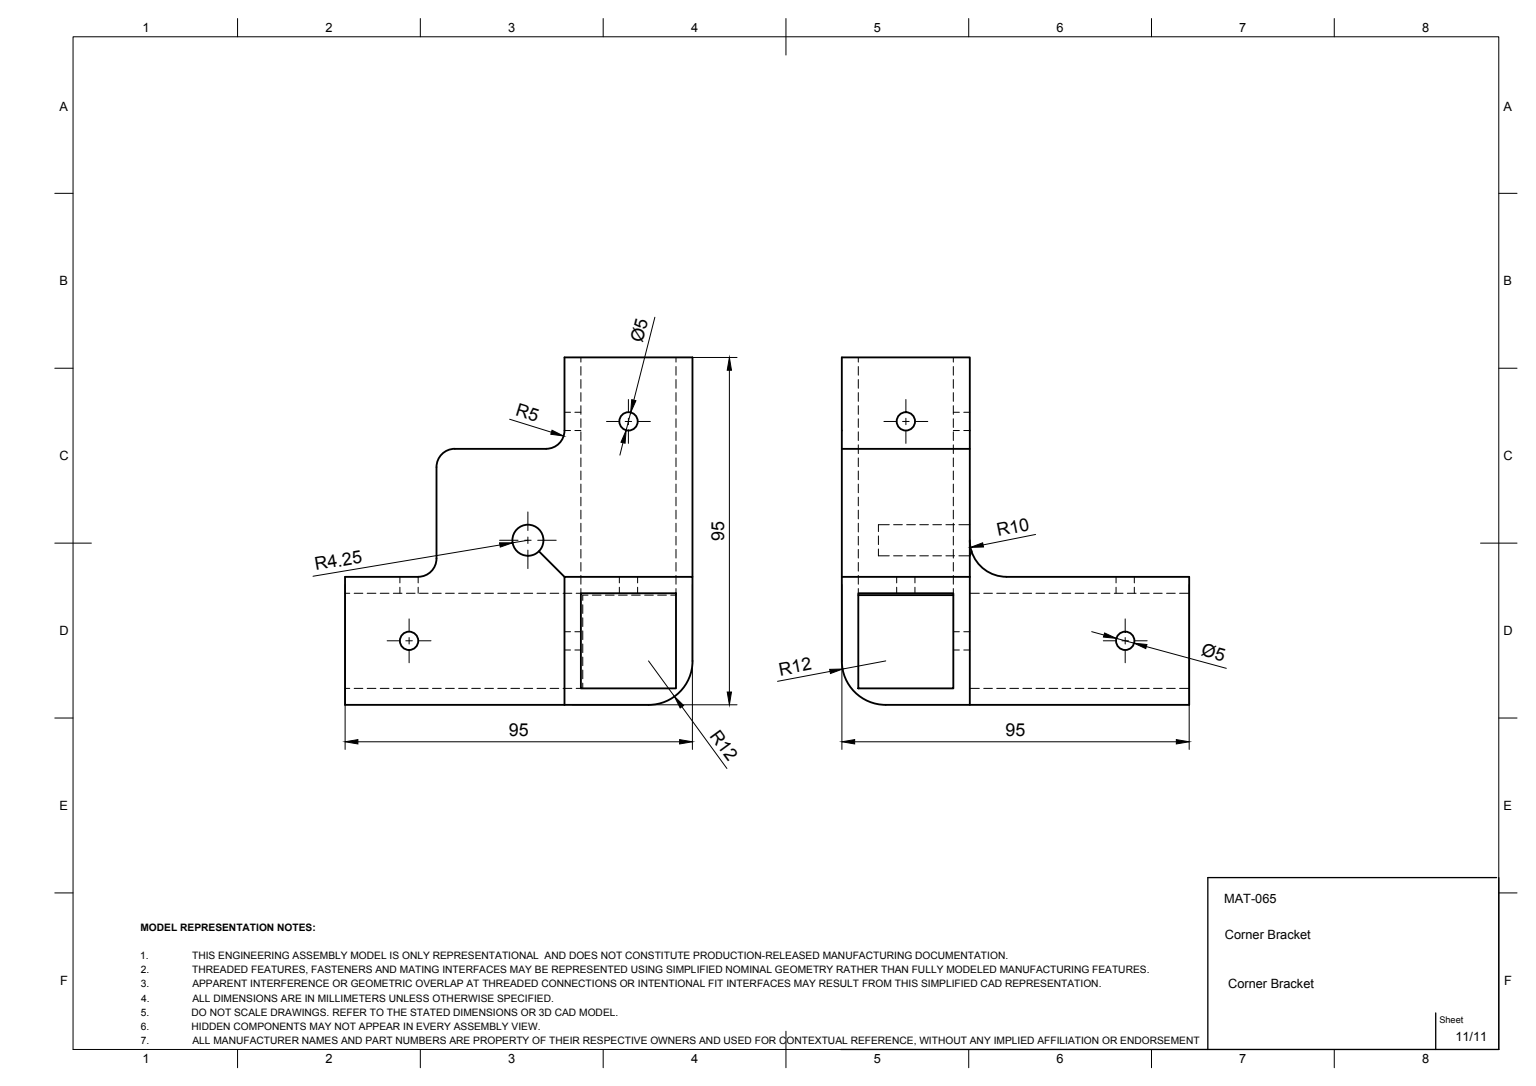
ISO-10303-21;
HEADER;
/* Generated by software containing ST-Developer
 * from STEP Tools, Inc. (www.steptools.com) 
 */

FILE_DESCRIPTION(
/* description */ (
'CAx-IF Rec.Pracs.---Representation and Presentation of Product Manufa
cturing Information (PMI)---4.0---2014-10-13'),
/* implementation_level */ '2;1');

FILE_NAME(
/* name */ 'Corner Bracket.step',
/* time_stamp */ '2026-11-15T23:28:27-08:00',
/* author */ (''),
/* organization */ (''),
/* preprocessor_version */ 'ST-DEVELOPER v20.2',
/* originating_system */ 'Autodesk Translation Framework v15.17.0.0',
/* authorisation */ '');

FILE_SCHEMA (('AUTOMOTIVE_DESIGN { 1 0 10303 214 3 1 1 }'));
ENDSEC;

DATA;
#10=MECHANICAL_DESIGN_GEOMETRIC_PRESENTATION_REPRESENTATION('',(#195),#7756);
#163=SPHERICAL_SURFACE('',#4954,0.012);
#165=ELLIPSE('',#4934,0.0141421356237309,0.01);
#167=B_SPLINE_CURVE_WITH_KNOTS('',3,(#7200,#7201,#7202,#7203,#7204,#7205),
 .UNSPECIFIED.,.F.,.F.,(4,2,4),(-0.973960746358264,-0.811705326326323,-0.649449906294381),
 .UNSPECIFIED.);
#168=B_SPLINE_CURVE_WITH_KNOTS('',3,(#7231,#7232,#7233,#7234,#7235,#7236),
 .UNSPECIFIED.,.F.,.F.,(4,2,4),(0.649449906294381,0.811705326326323,0.973960746358265),
 .UNSPECIFIED.);
#177=SHAPE_REPRESENTATION_RELATIONSHIP('SRR','None',#7825,#186);
#186=ADVANCED_BREP_SHAPE_REPRESENTATION('',(#204),#7753);
#195=STYLED_ITEM('',(#7873),#204);
#204=MANIFOLD_SOLID_BREP('Body1',#4632);
#224=CYLINDRICAL_SURFACE('',#4933,0.01);
#225=CYLINDRICAL_SURFACE('',#4935,0.012);
#226=CYLINDRICAL_SURFACE('',#4937,0.0025);
#227=CYLINDRICAL_SURFACE('',#4938,0.0025);
#228=CYLINDRICAL_SURFACE('',#4939,0.0025);
#229=CYLINDRICAL_SURFACE('',#4940,0.0025);
#230=CYLINDRICAL_SURFACE('',#4941,0.0025);
#231=CYLINDRICAL_SURFACE('',#4942,0.0025);
#232=CYLINDRICAL_SURFACE('',#4945,0.00425);
#233=CYLINDRICAL_SURFACE('',#4948,0.01);
#234=CYLINDRICAL_SURFACE('',#4949,0.005);
#235=CYLINDRICAL_SURFACE('',#4950,0.005);
#236=CYLINDRICAL_SURFACE('',#4951,0.005);
#237=CYLINDRICAL_SURFACE('',#4952,0.012);
#238=CYLINDRICAL_SURFACE('',#4956,0.012);
#298=CIRCLE('',#4884,0.0025);
#299=CIRCLE('',#4885,0.0025);
#300=CIRCLE('',#4887,0.0025);
#301=CIRCLE('',#4888,0.0025);
#302=CIRCLE('',#4890,0.012);
#303=CIRCLE('',#4892,0.012);
#304=CIRCLE('',#4895,0.012);
#305=CIRCLE('',#4897,0.01);
#306=CIRCLE('',#4899,0.01);
#307=CIRCLE('',#4901,0.005);
#308=CIRCLE('',#4902,0.005);
#309=CIRCLE('',#4903,0.00425);
#310=CIRCLE('',#4904,0.005);
#311=CIRCLE('',#4905,0.0025);
#312=CIRCLE('',#4906,0.0025);
#313=CIRCLE('',#4908,0.005);
#314=CIRCLE('',#4909,0.005);
#315=CIRCLE('',#4910,0.005);
#316=CIRCLE('',#4912,0.0025);
#317=CIRCLE('',#4914,0.0025);
#318=CIRCLE('',#4916,0.0025);
#319=CIRCLE('',#4917,0.0025);
#320=CIRCLE('',#4921,0.0025);
#321=CIRCLE('',#4923,0.0025);
#322=CIRCLE('',#4927,0.0025);
#323=CIRCLE('',#4931,0.0025);
#324=CIRCLE('',#4936,0.012);
#325=CIRCLE('',#4946,0.00425);
#326=CIRCLE('',#4953,0.012);
#327=CIRCLE('',#4955,0.012);
#407=FACE_BOUND('',#823,.T.);
#408=FACE_BOUND('',#825,.T.);
#409=FACE_BOUND('',#828,.T.);
#410=FACE_BOUND('',#832,.T.);
#411=FACE_BOUND('',#833,.T.);
#412=FACE_BOUND('',#836,.T.);
#413=FACE_BOUND('',#838,.T.);
#414=FACE_BOUND('',#840,.T.);
#415=FACE_BOUND('',#841,.T.);
#416=FACE_BOUND('',#845,.T.);
#417=FACE_BOUND('',#847,.T.);
#418=FACE_BOUND('',#851,.T.);
#419=FACE_BOUND('',#855,.T.);
#558=FACE_OUTER_BOUND('',#820,.T.);
#559=FACE_OUTER_BOUND('',#821,.T.);
#560=FACE_OUTER_BOUND('',#822,.T.);
#561=FACE_OUTER_BOUND('',#824,.T.);
#562=FACE_OUTER_BOUND('',#826,.T.);
#563=FACE_OUTER_BOUND('',#827,.T.);
#564=FACE_OUTER_BOUND('',#829,.T.);
#565=FACE_OUTER_BOUND('',#830,.T.);
#566=FACE_OUTER_BOUND('',#831,.T.);
#567=FACE_OUTER_BOUND('',#834,.T.);
#568=FACE_OUTER_BOUND('',#835,.T.);
#569=FACE_OUTER_BOUND('',#837,.T.);
#570=FACE_OUTER_BOUND('',#839,.T.);
#571=FACE_OUTER_BOUND('',#842,.T.);
#572=FACE_OUTER_BOUND('',#843,.T.);
#573=FACE_OUTER_BOUND('',#844,.T.);
#574=FACE_OUTER_BOUND('',#846,.T.);
#575=FACE_OUTER_BOUND('',#848,.T.);
#576=FACE_OUTER_BOUND('',#849,.T.);
#577=FACE_OUTER_BOUND('',#850,.T.);
#578=FACE_OUTER_BOUND('',#852,.T.);
#579=FACE_OUTER_BOUND('',#853,.T.);
#580=FACE_OUTER_BOUND('',#854,.T.);
#581=FACE_OUTER_BOUND('',#856,.T.);
#582=FACE_OUTER_BOUND('',#857,.T.);
#583=FACE_OUTER_BOUND('',#858,.T.);
#584=FACE_OUTER_BOUND('',#859,.T.);
#585=FACE_OUTER_BOUND('',#860,.T.);
#586=FACE_OUTER_BOUND('',#861,.T.);
#587=FACE_OUTER_BOUND('',#862,.T.);
#588=FACE_OUTER_BOUND('',#863,.T.);
#589=FACE_OUTER_BOUND('',#864,.T.);
#590=FACE_OUTER_BOUND('',#865,.T.);
#591=FACE_OUTER_BOUND('',#866,.T.);
#592=FACE_OUTER_BOUND('',#867,.T.);
#593=FACE_OUTER_BOUND('',#868,.T.);
#594=FACE_OUTER_BOUND('',#869,.T.);
#595=FACE_OUTER_BOUND('',#870,.T.);
#596=FACE_OUTER_BOUND('',#871,.T.);
#597=FACE_OUTER_BOUND('',#872,.T.);
#598=FACE_OUTER_BOUND('',#873,.T.);
#599=FACE_OUTER_BOUND('',#874,.T.);
#600=FACE_OUTER_BOUND('',#875,.T.);
#820=EDGE_LOOP('',(#3551,#3552,#3553,#3554,#3555,#3556,#3557));
#821=EDGE_LOOP('',(#3558,#3559,#3560,#3561,#3562,#3563,#3564));
#822=EDGE_LOOP('',(#3565,#3566,#3567,#3568,#3569));
#823=EDGE_LOOP('',(#3570,#3571,#3572,#3573));
#824=EDGE_LOOP('',(#3574,#3575,#3576,#3577,#3578));
#825=EDGE_LOOP('',(#3579,#3580,#3581,#3582));
#826=EDGE_LOOP('',(#3583,#3584,#3585,#3586));
#827=EDGE_LOOP('',(#3587,#3588,#3589,#3590,#3591));
#828=EDGE_LOOP('',(#3592,#3593,#3594,#3595));
#829=EDGE_LOOP('',(#3596,#3597,#3598,#3599,#3600,#3601,#3602));
#830=EDGE_LOOP('',(#3603,#3604,#3605,#3606,#3607,#3608,#3609));
#831=EDGE_LOOP('',(#3610,#3611,#3612,#3613,#3614,#3615,#3616,#3617,#3618,
#3619,#3620,#3621,#3622,#3623));
#832=EDGE_LOOP('',(#3624));
#833=EDGE_LOOP('',(#3625));
#834=EDGE_LOOP('',(#3626,#3627,#3628,#3629,#3630,#3631,#3632,#3633,#3634,
#3635,#3636));
#835=EDGE_LOOP('',(#3637,#3638,#3639,#3640));
#836=EDGE_LOOP('',(#3641));
#837=EDGE_LOOP('',(#3642,#3643,#3644,#3645));
#838=EDGE_LOOP('',(#3646));
#839=EDGE_LOOP('',(#3647,#3648,#3649,#3650,#3651,#3652,#3653,#3654));
#840=EDGE_LOOP('',(#3655));
#841=EDGE_LOOP('',(#3656));
#842=EDGE_LOOP('',(#3657,#3658,#3659,#3660));
#843=EDGE_LOOP('',(#3661,#3662,#3663,#3664,#3665,#3666,#3667,#3668));
#844=EDGE_LOOP('',(#3669,#3670,#3671,#3672));
#845=EDGE_LOOP('',(#3673));
#846=EDGE_LOOP('',(#3674,#3675,#3676,#3677));
#847=EDGE_LOOP('',(#3678));
#848=EDGE_LOOP('',(#3679,#3680,#3681,#3682));
#849=EDGE_LOOP('',(#3683,#3684,#3685,#3686));
#850=EDGE_LOOP('',(#3687,#3688,#3689,#3690));
#851=EDGE_LOOP('',(#3691));
#852=EDGE_LOOP('',(#3692,#3693,#3694,#3695));
#853=EDGE_LOOP('',(#3696,#3697,#3698,#3699));
#854=EDGE_LOOP('',(#3700,#3701,#3702,#3703));
#855=EDGE_LOOP('',(#3704));
#856=EDGE_LOOP('',(#3705,#3706,#3707,#3708));
#857=EDGE_LOOP('',(#3709,#3710,#3711,#3712,#3713));
#858=EDGE_LOOP('',(#3714,#3715,#3716,#3717));
#859=EDGE_LOOP('',(#3718,#3719,#3720,#3721));
#860=EDGE_LOOP('',(#3722,#3723,#3724,#3725));
#861=EDGE_LOOP('',(#3726,#3727,#3728,#3729));
#862=EDGE_LOOP('',(#3730,#3731,#3732,#3733,#3734));
#863=EDGE_LOOP('',(#3735,#3736,#3737,#3738));
#864=EDGE_LOOP('',(#3739,#3740,#3741,#3742,#3743));
#865=EDGE_LOOP('',(#3744,#3745,#3746,#3747));
#866=EDGE_LOOP('',(#3748,#3749,#3750,#3751));
#867=EDGE_LOOP('',(#3752,#3753,#3754,#3755,#3756,#3757));
#868=EDGE_LOOP('',(#3758));
#869=EDGE_LOOP('',(#3759,#3760,#3761,#3762,#3763));
#870=EDGE_LOOP('',(#3764,#3765,#3766,#3767,#3768));
#871=EDGE_LOOP('',(#3769,#3770,#3771,#3772,#3773));
#872=EDGE_LOOP('',(#3774,#3775,#3776,#3777));
#873=EDGE_LOOP('',(#3778,#3779,#3780,#3781));
#874=EDGE_LOOP('',(#3782,#3783,#3784));
#875=EDGE_LOOP('',(#3785,#3786,#3787,#3788));
#1237=LINE('',#7001,#1730);
#1238=LINE('',#7003,#1731);
#1239=LINE('',#7008,#1732);
#1240=LINE('',#7010,#1733);
#1241=LINE('',#7011,#1734);
#1242=LINE('',#7015,#1735);
#1243=LINE('',#7017,#1736);
#1244=LINE('',#7022,#1737);
#1245=LINE('',#7024,#1738);
#1246=LINE('',#7025,#1739);
#1247=LINE('',#7029,#1740);
#1248=LINE('',#7033,#1741);
#1249=LINE('',#7035,#1742);
#1250=LINE('',#7036,#1743);
#1251=LINE('',#7039,#1744);
#1252=LINE('',#7041,#1745);
#1253=LINE('',#7043,#1746);
#1254=LINE('',#7044,#1747);
#1255=LINE('',#7047,#1748);
#1256=LINE('',#7051,#1749);
#1257=LINE('',#7052,#1750);
#1258=LINE('',#7055,#1751);
#1259=LINE('',#7057,#1752);
#1260=LINE('',#7059,#1753);
#1261=LINE('',#7060,#1754);
#1262=LINE('',#7064,#1755);
#1263=LINE('',#7066,#1756);
#1264=LINE('',#7068,#1757);
#1265=LINE('',#7069,#1758);
#1266=LINE('',#7073,#1759);
#1267=LINE('',#7076,#1760);
#1268=LINE('',#7077,#1761);
#1269=LINE('',#7080,#1762);
#1270=LINE('',#7082,#1763);
#1271=LINE('',#7084,#1764);
#1272=LINE('',#7085,#1765);
#1273=LINE('',#7088,#1766);
#1274=LINE('',#7089,#1767);
#1275=LINE('',#7091,#1768);
#1276=LINE('',#7094,#1769);
#1277=LINE('',#7097,#1770);
#1278=LINE('',#7098,#1771);
#1279=LINE('',#7100,#1772);
#1280=LINE('',#7103,#1773);
#1281=LINE('',#7107,#1774);
#1282=LINE('',#7111,#1775);
#1283=LINE('',#7114,#1776);
#1284=LINE('',#7117,#1777);
#1285=LINE('',#7125,#1778);
#1286=LINE('',#7126,#1779);
#1287=LINE('',#7130,#1780);
#1288=LINE('',#7134,#1781);
#1289=LINE('',#7138,#1782);
#1290=LINE('',#7139,#1783);
#1291=LINE('',#7143,#1784);
#1292=LINE('',#7148,#1785);
#1293=LINE('',#7149,#1786);
#1294=LINE('',#7151,#1787);
#1295=LINE('',#7152,#1788);
#1296=LINE('',#7153,#1789);
#1297=LINE('',#7159,#1790);
#1298=LINE('',#7162,#1791);
#1299=LINE('',#7163,#1792);
#1300=LINE('',#7165,#1793);
#1301=LINE('',#7166,#1794);
#1302=LINE('',#7168,#1795);
#1303=LINE('',#7175,#1796);
#1304=LINE('',#7179,#1797);
#1305=LINE('',#7181,#1798);
#1306=LINE('',#7182,#1799);
#1307=LINE('',#7187,#1800);
#1308=LINE('',#7188,#1801);
#1309=LINE('',#7191,#1802);
#1310=LINE('',#7192,#1803);
#1311=LINE('',#7194,#1804);
#1312=LINE('',#7210,#1805);
#1313=LINE('',#7212,#1806);
#1314=LINE('',#7214,#1807);
#1315=LINE('',#7216,#1808);
#1316=LINE('',#7218,#1809);
#1317=LINE('',#7220,#1810);
#1318=LINE('',#7222,#1811);
#1319=LINE('',#7223,#1812);
#1320=LINE('',#7225,#1813);
#1321=LINE('',#7226,#1814);
#1322=LINE('',#7230,#1815);
#1730=VECTOR('',#5675,1.);
#1731=VECTOR('',#5676,1.);
#1732=VECTOR('',#5681,1.);
#1733=VECTOR('',#5682,1.);
#1734=VECTOR('',#5683,1.);
#1735=VECTOR('',#5686,1.);
#1736=VECTOR('',#5687,1.);
#1737=VECTOR('',#5692,1.);
#1738=VECTOR('',#5693,1.);
#1739=VECTOR('',#5694,1.);
#1740=VECTOR('',#5697,1.);
#1741=VECTOR('',#5700,1.);
#1742=VECTOR('',#5701,1.);
#1743=VECTOR('',#5702,1.);
#1744=VECTOR('',#5703,1.);
#1745=VECTOR('',#5704,1.);
#1746=VECTOR('',#5705,1.);
#1747=VECTOR('',#5706,1.);
#1748=VECTOR('',#5709,1.);
#1749=VECTOR('',#5712,1.);
#1750=VECTOR('',#5713,1.);
#1751=VECTOR('',#5714,1.);
#1752=VECTOR('',#5715,1.);
#1753=VECTOR('',#5716,1.);
#1754=VECTOR('',#5717,1.);
#1755=VECTOR('',#5720,1.);
#1756=VECTOR('',#5721,1.);
#1757=VECTOR('',#5722,1.);
#1758=VECTOR('',#5723,1.);
#1759=VECTOR('',#5726,1.);
#1760=VECTOR('',#5729,1.);
#1761=VECTOR('',#5730,1.);
#1762=VECTOR('',#5731,1.);
#1763=VECTOR('',#5732,1.);
#1764=VECTOR('',#5733,1.);
#1765=VECTOR('',#5734,1.);
#1766=VECTOR('',#5737,1.);
#1767=VECTOR('',#5738,1.);
#1768=VECTOR('',#5739,1.);
#1769=VECTOR('',#5742,1.);
#1770=VECTOR('',#5745,1.);
#1771=VECTOR('',#5746,1.);
#1772=VECTOR('',#5747,1.);
#1773=VECTOR('',#5750,1.);
#1774=VECTOR('',#5753,1.);
#1775=VECTOR('',#5756,1.);
#1776=VECTOR('',#5759,1.);
#1777=VECTOR('',#5762,1.);
#1778=VECTOR('',#5771,1.);
#1779=VECTOR('',#5772,1.);
#1780=VECTOR('',#5775,1.);
#1781=VECTOR('',#5778,1.);
#1782=VECTOR('',#5783,1.);
#1783=VECTOR('',#5784,1.);
#1784=VECTOR('',#5789,1.);
#1785=VECTOR('',#5794,1.);
#1786=VECTOR('',#5795,1.);
#1787=VECTOR('',#5796,1.);
#1788=VECTOR('',#5797,1.);
#1789=VECTOR('',#5798,1.);
#1790=VECTOR('',#5805,1.);
#1791=VECTOR('',#5808,1.);
#1792=VECTOR('',#5809,1.);
#1793=VECTOR('',#5810,1.);
#1794=VECTOR('',#5811,1.);
#1795=VECTOR('',#5814,1.);
#1796=VECTOR('',#5823,1.);
#1797=VECTOR('',#5828,1.);
#1798=VECTOR('',#5829,1.);
#1799=VECTOR('',#5830,1.);
#1800=VECTOR('',#5835,1.);
#1801=VECTOR('',#5836,1.);
#1802=VECTOR('',#5839,1.);
#1803=VECTOR('',#5840,1.);
#1804=VECTOR('',#5843,1.);
#1805=VECTOR('',#5858,0.0025);
#1806=VECTOR('',#5861,0.0025);
#1807=VECTOR('',#5864,0.0025);
#1808=VECTOR('',#5867,0.0025);
#1809=VECTOR('',#5870,0.0025);
#1810=VECTOR('',#5873,0.0025);
#1811=VECTOR('',#5876,1.);
#1812=VECTOR('',#5877,1.);
#1813=VECTOR('',#5880,1.);
#1814=VECTOR('',#5881,1.);
#1815=VECTOR('',#5886,0.00425);
#2164=VERTEX_POINT('',#6999);
#2165=VERTEX_POINT('',#7000);
#2166=VERTEX_POINT('',#7002);
#2167=VERTEX_POINT('',#7004);
#2168=VERTEX_POINT('',#7007);
#2169=VERTEX_POINT('',#7009);
#2170=VERTEX_POINT('',#7013);
#2171=VERTEX_POINT('',#7014);
#2172=VERTEX_POINT('',#7016);
#2173=VERTEX_POINT('',#7018);
#2174=VERTEX_POINT('',#7021);
#2175=VERTEX_POINT('',#7023);
#2176=VERTEX_POINT('',#7027);
#2177=VERTEX_POINT('',#7028);
#2178=VERTEX_POINT('',#7030);
#2179=VERTEX_POINT('',#7032);
#2180=VERTEX_POINT('',#7034);
#2181=VERTEX_POINT('',#7037);
#2182=VERTEX_POINT('',#7038);
#2183=VERTEX_POINT('',#7040);
#2184=VERTEX_POINT('',#7042);
#2185=VERTEX_POINT('',#7046);
#2186=VERTEX_POINT('',#7048);
#2187=VERTEX_POINT('',#7050);
#2188=VERTEX_POINT('',#7053);
#2189=VERTEX_POINT('',#7054);
#2190=VERTEX_POINT('',#7056);
#2191=VERTEX_POINT('',#7058);
#2192=VERTEX_POINT('',#7062);
#2193=VERTEX_POINT('',#7063);
#2194=VERTEX_POINT('',#7065);
#2195=VERTEX_POINT('',#7067);
#2196=VERTEX_POINT('',#7071);
#2197=VERTEX_POINT('',#7072);
#2198=VERTEX_POINT('',#7074);
#2199=VERTEX_POINT('',#7078);
#2200=VERTEX_POINT('',#7079);
#2201=VERTEX_POINT('',#7081);
#2202=VERTEX_POINT('',#7083);
#2203=VERTEX_POINT('',#7087);
#2204=VERTEX_POINT('',#7090);
#2205=VERTEX_POINT('',#7092);
#2206=VERTEX_POINT('',#7096);
#2207=VERTEX_POINT('',#7099);
#2208=VERTEX_POINT('',#7101);
#2209=VERTEX_POINT('',#7105);
#2210=VERTEX_POINT('',#7106);
#2211=VERTEX_POINT('',#7108);
#2212=VERTEX_POINT('',#7110);
#2213=VERTEX_POINT('',#7113);
#2214=VERTEX_POINT('',#7115);
#2215=VERTEX_POINT('',#7119);
#2216=VERTEX_POINT('',#7121);
#2217=VERTEX_POINT('',#7124);
#2218=VERTEX_POINT('',#7127);
#2219=VERTEX_POINT('',#7129);
#2220=VERTEX_POINT('',#7131);
#2221=VERTEX_POINT('',#7133);
#2222=VERTEX_POINT('',#7137);
#2223=VERTEX_POINT('',#7140);
#2224=VERTEX_POINT('',#7144);
#2225=VERTEX_POINT('',#7147);
#2226=VERTEX_POINT('',#7150);
#2227=VERTEX_POINT('',#7154);
#2228=VERTEX_POINT('',#7156);
#2229=VERTEX_POINT('',#7161);
#2230=VERTEX_POINT('',#7164);
#2231=VERTEX_POINT('',#7169);
#2232=VERTEX_POINT('',#7172);
#2233=VERTEX_POINT('',#7178);
#2234=VERTEX_POINT('',#7180);
#2235=VERTEX_POINT('',#7183);
#2236=VERTEX_POINT('',#7186);
#2237=VERTEX_POINT('',#7190);
#2238=VERTEX_POINT('',#7195);
#2239=VERTEX_POINT('',#7199);
#2240=VERTEX_POINT('',#7228);
#2659=EDGE_CURVE('',#2164,#2165,#1237,.T.);
#2660=EDGE_CURVE('',#2165,#2166,#1238,.T.);
#2661=EDGE_CURVE('',#2167,#2166,#298,.T.);
#2662=EDGE_CURVE('',#2166,#2167,#299,.T.);
#2663=EDGE_CURVE('',#2166,#2168,#1239,.T.);
#2664=EDGE_CURVE('',#2169,#2168,#1240,.T.);
#2665=EDGE_CURVE('',#2164,#2169,#1241,.T.);
#2666=EDGE_CURVE('',#2170,#2171,#1242,.T.);
#2667=EDGE_CURVE('',#2170,#2172,#1243,.F.);
#2668=EDGE_CURVE('',#2173,#2172,#300,.T.);
#2669=EDGE_CURVE('',#2172,#2173,#301,.T.);
#2670=EDGE_CURVE('',#2172,#2174,#1244,.F.);
#2671=EDGE_CURVE('',#2174,#2175,#1245,.T.);
#2672=EDGE_CURVE('',#2175,#2171,#1246,.T.);
#2673=EDGE_CURVE('',#2176,#2177,#1247,.T.);
#2674=EDGE_CURVE('',#2177,#2178,#302,.T.);
#2675=EDGE_CURVE('',#2178,#2179,#1248,.T.);
#2676=EDGE_CURVE('',#2180,#2179,#1249,.T.);
#2677=EDGE_CURVE('',#2180,#2176,#1250,.T.);
#2678=EDGE_CURVE('',#2181,#2182,#1251,.T.);
#2679=EDGE_CURVE('',#2181,#2183,#1252,.T.);
#2680=EDGE_CURVE('',#2183,#2184,#1253,.T.);
#2681=EDGE_CURVE('',#2182,#2184,#1254,.T.);
#2682=EDGE_CURVE('',#2185,#2169,#1255,.T.);
#2683=EDGE_CURVE('',#2185,#2186,#303,.T.);
#2684=EDGE_CURVE('',#2187,#2186,#1256,.T.);
#2685=EDGE_CURVE('',#2187,#2164,#1257,.T.);
#2686=EDGE_CURVE('',#2188,#2189,#1258,.T.);
#2687=EDGE_CURVE('',#2188,#2190,#1259,.T.);
#2688=EDGE_CURVE('',#2190,#2191,#1260,.T.);
#2689=EDGE_CURVE('',#2189,#2191,#1261,.T.);
#2690=EDGE_CURVE('',#2192,#2193,#1262,.T.);
#2691=EDGE_CURVE('',#2193,#2194,#1263,.T.);
#2692=EDGE_CURVE('',#2195,#2194,#1264,.T.);
#2693=EDGE_CURVE('',#2195,#2192,#1265,.T.);
#2694=EDGE_CURVE('',#2196,#2197,#1266,.T.);
#2695=EDGE_CURVE('',#2197,#2198,#304,.T.);
#2696=EDGE_CURVE('',#2171,#2198,#1267,.T.);
#2697=EDGE_CURVE('',#2175,#2196,#1268,.T.);
#2698=EDGE_CURVE('',#2199,#2200,#1269,.T.);
#2699=EDGE_CURVE('',#2199,#2201,#1270,.T.);
#2700=EDGE_CURVE('',#2201,#2202,#1271,.T.);
#2701=EDGE_CURVE('',#2200,#2202,#1272,.T.);
#2702=EDGE_CURVE('',#2186,#2203,#1273,.T.);
#2703=EDGE_CURVE('',#2203,#2177,#1274,.F.);
#2704=EDGE_CURVE('',#2176,#2204,#1275,.T.);
#2705=EDGE_CURVE('',#2204,#2205,#305,.T.);
#2706=EDGE_CURVE('',#2187,#2205,#1276,.T.);
#2707=EDGE_CURVE('',#2178,#2206,#1277,.T.);
#2708=EDGE_CURVE('',#2206,#2197,#1278,.T.);
#2709=EDGE_CURVE('',#2207,#2196,#1279,.T.);
#2710=EDGE_CURVE('',#2207,#2208,#306,.T.);
#2711=EDGE_CURVE('',#2179,#2208,#1280,.T.);
#2712=EDGE_CURVE('',#2209,#2210,#1281,.T.);
#2713=EDGE_CURVE('',#2209,#2211,#307,.T.);
#2714=EDGE_CURVE('',#2211,#2212,#1282,.T.);
#2715=EDGE_CURVE('',#2212,#2165,#308,.F.);
#2716=EDGE_CURVE('',#2205,#2213,#1283,.F.);
#2717=EDGE_CURVE('',#2214,#2213,#309,.T.);
#2718=EDGE_CURVE('',#2214,#2207,#1284,.T.);
#2719=EDGE_CURVE('',#2174,#2210,#310,.F.);
#2720=EDGE_CURVE('',#2215,#2215,#311,.T.);
#2721=EDGE_CURVE('',#2216,#2216,#312,.T.);
#2722=EDGE_CURVE('',#2198,#2217,#1285,.F.);
#2723=EDGE_CURVE('',#2217,#2185,#1286,.F.);
#2724=EDGE_CURVE('',#2168,#2218,#313,.T.);
#2725=EDGE_CURVE('',#2219,#2218,#1287,.T.);
#2726=EDGE_CURVE('',#2219,#2220,#314,.F.);
#2727=EDGE_CURVE('',#2220,#2221,#1288,.T.);
#2728=EDGE_CURVE('',#2221,#2170,#315,.T.);
#2729=EDGE_CURVE('',#2208,#2222,#1289,.F.);
#2730=EDGE_CURVE('',#2180,#2222,#1290,.T.);
#2731=EDGE_CURVE('',#2223,#2223,#316,.T.);
#2732=EDGE_CURVE('',#2222,#2204,#1291,.T.);
#2733=EDGE_CURVE('',#2224,#2224,#317,.T.);
#2734=EDGE_CURVE('',#2194,#2225,#1292,.T.);
#2735=EDGE_CURVE('',#2225,#2190,#1293,.T.);
#2736=EDGE_CURVE('',#2226,#2188,#1294,.T.);
#2737=EDGE_CURVE('',#2226,#2201,#1295,.T.);
#2738=EDGE_CURVE('',#2195,#2199,#1296,.T.);
#2739=EDGE_CURVE('',#2227,#2227,#318,.T.);
#2740=EDGE_CURVE('',#2228,#2228,#319,.T.);
#2741=EDGE_CURVE('',#2192,#2200,#1297,.T.);
#2742=EDGE_CURVE('',#2229,#2202,#1298,.T.);
#2743=EDGE_CURVE('',#2229,#2189,#1299,.T.);
#2744=EDGE_CURVE('',#2230,#2191,#1300,.T.);
#2745=EDGE_CURVE('',#2193,#2230,#1301,.T.);
#2746=EDGE_CURVE('',#2229,#2226,#1302,.T.);
#2747=EDGE_CURVE('',#2231,#2231,#320,.T.);
#2748=EDGE_CURVE('',#2232,#2232,#321,.T.);
#2749=EDGE_CURVE('',#2225,#2230,#1303,.T.);
#2750=EDGE_CURVE('',#2233,#2181,#1304,.T.);
#2751=EDGE_CURVE('',#2233,#2234,#1305,.T.);
#2752=EDGE_CURVE('',#2234,#2183,#1306,.T.);
#2753=EDGE_CURVE('',#2235,#2235,#322,.T.);
#2754=EDGE_CURVE('',#2236,#2182,#1307,.T.);
#2755=EDGE_CURVE('',#2233,#2236,#1308,.T.);
#2756=EDGE_CURVE('',#2237,#2184,#1309,.T.);
#2757=EDGE_CURVE('',#2236,#2237,#1310,.T.);
#2758=EDGE_CURVE('',#2234,#2237,#1311,.T.);
#2759=EDGE_CURVE('',#2238,#2238,#323,.T.);
#2760=EDGE_CURVE('',#2214,#2239,#167,.F.);
#2761=EDGE_CURVE('',#2239,#2222,#165,.T.);
#2762=EDGE_CURVE('',#2203,#2206,#324,.F.);
#2763=EDGE_CURVE('',#2228,#2216,#1312,.T.);
#2764=EDGE_CURVE('',#2227,#2215,#1313,.T.);
#2765=EDGE_CURVE('',#2235,#2224,#1314,.T.);
#2766=EDGE_CURVE('',#2231,#2173,#1315,.T.);
#2767=EDGE_CURVE('',#2238,#2223,#1316,.T.);
#2768=EDGE_CURVE('',#2232,#2167,#1317,.T.);
#2769=EDGE_CURVE('',#2218,#2212,#1318,.F.);
#2770=EDGE_CURVE('',#2211,#2219,#1319,.T.);
#2771=EDGE_CURVE('',#2210,#2221,#1320,.T.);
#2772=EDGE_CURVE('',#2220,#2209,#1321,.F.);
#2773=EDGE_CURVE('',#2240,#2240,#325,.T.);
#2774=EDGE_CURVE('',#2240,#2213,#1322,.T.);
#2775=EDGE_CURVE('',#2213,#2239,#168,.T.);
#2776=EDGE_CURVE('',#2217,#2206,#326,.T.);
#2777=EDGE_CURVE('',#2217,#2203,#327,.T.);
#3551=ORIENTED_EDGE('',*,*,#2659,.T.);
#3552=ORIENTED_EDGE('',*,*,#2660,.T.);
#3553=ORIENTED_EDGE('',*,*,#2661,.F.);
#3554=ORIENTED_EDGE('',*,*,#2662,.F.);
#3555=ORIENTED_EDGE('',*,*,#2663,.T.);
#3556=ORIENTED_EDGE('',*,*,#2664,.F.);
#3557=ORIENTED_EDGE('',*,*,#2665,.F.);
#3558=ORIENTED_EDGE('',*,*,#2666,.F.);
#3559=ORIENTED_EDGE('',*,*,#2667,.T.);
#3560=ORIENTED_EDGE('',*,*,#2668,.F.);
#3561=ORIENTED_EDGE('',*,*,#2669,.F.);
#3562=ORIENTED_EDGE('',*,*,#2670,.T.);
#3563=ORIENTED_EDGE('',*,*,#2671,.T.);
#3564=ORIENTED_EDGE('',*,*,#2672,.T.);
#3565=ORIENTED_EDGE('',*,*,#2673,.T.);
#3566=ORIENTED_EDGE('',*,*,#2674,.T.);
#3567=ORIENTED_EDGE('',*,*,#2675,.T.);
#3568=ORIENTED_EDGE('',*,*,#2676,.F.);
#3569=ORIENTED_EDGE('',*,*,#2677,.T.);
#3570=ORIENTED_EDGE('',*,*,#2678,.F.);
#3571=ORIENTED_EDGE('',*,*,#2679,.T.);
#3572=ORIENTED_EDGE('',*,*,#2680,.T.);
#3573=ORIENTED_EDGE('',*,*,#2681,.F.);
#3574=ORIENTED_EDGE('',*,*,#2682,.F.);
#3575=ORIENTED_EDGE('',*,*,#2683,.T.);
#3576=ORIENTED_EDGE('',*,*,#2684,.F.);
#3577=ORIENTED_EDGE('',*,*,#2685,.T.);
#3578=ORIENTED_EDGE('',*,*,#2665,.T.);
#3579=ORIENTED_EDGE('',*,*,#2686,.F.);
#3580=ORIENTED_EDGE('',*,*,#2687,.T.);
#3581=ORIENTED_EDGE('',*,*,#2688,.T.);
#3582=ORIENTED_EDGE('',*,*,#2689,.F.);
#3583=ORIENTED_EDGE('',*,*,#2690,.T.);
#3584=ORIENTED_EDGE('',*,*,#2691,.T.);
#3585=ORIENTED_EDGE('',*,*,#2692,.F.);
#3586=ORIENTED_EDGE('',*,*,#2693,.T.);
#3587=ORIENTED_EDGE('',*,*,#2694,.T.);
#3588=ORIENTED_EDGE('',*,*,#2695,.T.);
#3589=ORIENTED_EDGE('',*,*,#2696,.F.);
#3590=ORIENTED_EDGE('',*,*,#2672,.F.);
#3591=ORIENTED_EDGE('',*,*,#2697,.T.);
#3592=ORIENTED_EDGE('',*,*,#2698,.F.);
#3593=ORIENTED_EDGE('',*,*,#2699,.T.);
#3594=ORIENTED_EDGE('',*,*,#2700,.T.);
#3595=ORIENTED_EDGE('',*,*,#2701,.F.);
#3596=ORIENTED_EDGE('',*,*,#2684,.T.);
#3597=ORIENTED_EDGE('',*,*,#2702,.T.);
#3598=ORIENTED_EDGE('',*,*,#2703,.T.);
#3599=ORIENTED_EDGE('',*,*,#2673,.F.);
#3600=ORIENTED_EDGE('',*,*,#2704,.T.);
#3601=ORIENTED_EDGE('',*,*,#2705,.T.);
#3602=ORIENTED_EDGE('',*,*,#2706,.F.);
#3603=ORIENTED_EDGE('',*,*,#2707,.T.);
#3604=ORIENTED_EDGE('',*,*,#2708,.T.);
#3605=ORIENTED_EDGE('',*,*,#2694,.F.);
#3606=ORIENTED_EDGE('',*,*,#2709,.F.);
#3607=ORIENTED_EDGE('',*,*,#2710,.T.);
#3608=ORIENTED_EDGE('',*,*,#2711,.F.);
#3609=ORIENTED_EDGE('',*,*,#2675,.F.);
#3610=ORIENTED_EDGE('',*,*,#2712,.F.);
#3611=ORIENTED_EDGE('',*,*,#2713,.T.);
#3612=ORIENTED_EDGE('',*,*,#2714,.T.);
#3613=ORIENTED_EDGE('',*,*,#2715,.T.);
#3614=ORIENTED_EDGE('',*,*,#2659,.F.);
#3615=ORIENTED_EDGE('',*,*,#2685,.F.);
#3616=ORIENTED_EDGE('',*,*,#2706,.T.);
#3617=ORIENTED_EDGE('',*,*,#2716,.T.);
#3618=ORIENTED_EDGE('',*,*,#2717,.F.);
#3619=ORIENTED_EDGE('',*,*,#2718,.T.);
#3620=ORIENTED_EDGE('',*,*,#2709,.T.);
#3621=ORIENTED_EDGE('',*,*,#2697,.F.);
#3622=ORIENTED_EDGE('',*,*,#2671,.F.);
#3623=ORIENTED_EDGE('',*,*,#2719,.T.);
#3624=ORIENTED_EDGE('',*,*,#2720,.F.);
#3625=ORIENTED_EDGE('',*,*,#2721,.F.);
#3626=ORIENTED_EDGE('',*,*,#2722,.T.);
#3627=ORIENTED_EDGE('',*,*,#2723,.T.);
#3628=ORIENTED_EDGE('',*,*,#2682,.T.);
#3629=ORIENTED_EDGE('',*,*,#2664,.T.);
#3630=ORIENTED_EDGE('',*,*,#2724,.T.);
#3631=ORIENTED_EDGE('',*,*,#2725,.F.);
#3632=ORIENTED_EDGE('',*,*,#2726,.T.);
#3633=ORIENTED_EDGE('',*,*,#2727,.T.);
#3634=ORIENTED_EDGE('',*,*,#2728,.T.);
#3635=ORIENTED_EDGE('',*,*,#2666,.T.);
#3636=ORIENTED_EDGE('',*,*,#2696,.T.);
#3637=ORIENTED_EDGE('',*,*,#2711,.T.);
#3638=ORIENTED_EDGE('',*,*,#2729,.T.);
#3639=ORIENTED_EDGE('',*,*,#2730,.F.);
#3640=ORIENTED_EDGE('',*,*,#2676,.T.);
#3641=ORIENTED_EDGE('',*,*,#2731,.F.);
#3642=ORIENTED_EDGE('',*,*,#2730,.T.);
#3643=ORIENTED_EDGE('',*,*,#2732,.T.);
#3644=ORIENTED_EDGE('',*,*,#2704,.F.);
#3645=ORIENTED_EDGE('',*,*,#2677,.F.);
#3646=ORIENTED_EDGE('',*,*,#2733,.F.);
#3647=ORIENTED_EDGE('',*,*,#2692,.T.);
#3648=ORIENTED_EDGE('',*,*,#2734,.T.);
#3649=ORIENTED_EDGE('',*,*,#2735,.T.);
#3650=ORIENTED_EDGE('',*,*,#2687,.F.);
#3651=ORIENTED_EDGE('',*,*,#2736,.F.);
#3652=ORIENTED_EDGE('',*,*,#2737,.T.);
#3653=ORIENTED_EDGE('',*,*,#2699,.F.);
#3654=ORIENTED_EDGE('',*,*,#2738,.F.);
#3655=ORIENTED_EDGE('',*,*,#2739,.F.);
#3656=ORIENTED_EDGE('',*,*,#2740,.F.);
#3657=ORIENTED_EDGE('',*,*,#2698,.T.);
#3658=ORIENTED_EDGE('',*,*,#2741,.F.);
#3659=ORIENTED_EDGE('',*,*,#2693,.F.);
#3660=ORIENTED_EDGE('',*,*,#2738,.T.);
#3661=ORIENTED_EDGE('',*,*,#2742,.F.);
#3662=ORIENTED_EDGE('',*,*,#2743,.T.);
#3663=ORIENTED_EDGE('',*,*,#2689,.T.);
#3664=ORIENTED_EDGE('',*,*,#2744,.F.);
#3665=ORIENTED_EDGE('',*,*,#2745,.F.);
#3666=ORIENTED_EDGE('',*,*,#2690,.F.);
#3667=ORIENTED_EDGE('',*,*,#2741,.T.);
#3668=ORIENTED_EDGE('',*,*,#2701,.T.);
#3669=ORIENTED_EDGE('',*,*,#2746,.F.);
#3670=ORIENTED_EDGE('',*,*,#2742,.T.);
#3671=ORIENTED_EDGE('',*,*,#2700,.F.);
#3672=ORIENTED_EDGE('',*,*,#2737,.F.);
#3673=ORIENTED_EDGE('',*,*,#2747,.F.);
#3674=ORIENTED_EDGE('',*,*,#2746,.T.);
#3675=ORIENTED_EDGE('',*,*,#2736,.T.);
#3676=ORIENTED_EDGE('',*,*,#2686,.T.);
#3677=ORIENTED_EDGE('',*,*,#2743,.F.);
#3678=ORIENTED_EDGE('',*,*,#2748,.T.);
#3679=ORIENTED_EDGE('',*,*,#2688,.F.);
#3680=ORIENTED_EDGE('',*,*,#2735,.F.);
#3681=ORIENTED_EDGE('',*,*,#2749,.T.);
#3682=ORIENTED_EDGE('',*,*,#2744,.T.);
#3683=ORIENTED_EDGE('',*,*,#2745,.T.);
#3684=ORIENTED_EDGE('',*,*,#2749,.F.);
#3685=ORIENTED_EDGE('',*,*,#2734,.F.);
#3686=ORIENTED_EDGE('',*,*,#2691,.F.);
#3687=ORIENTED_EDGE('',*,*,#2679,.F.);
#3688=ORIENTED_EDGE('',*,*,#2750,.F.);
#3689=ORIENTED_EDGE('',*,*,#2751,.T.);
#3690=ORIENTED_EDGE('',*,*,#2752,.T.);
#3691=ORIENTED_EDGE('',*,*,#2753,.F.);
#3692=ORIENTED_EDGE('',*,*,#2678,.T.);
#3693=ORIENTED_EDGE('',*,*,#2754,.F.);
#3694=ORIENTED_EDGE('',*,*,#2755,.F.);
#3695=ORIENTED_EDGE('',*,*,#2750,.T.);
#3696=ORIENTED_EDGE('',*,*,#2681,.T.);
#3697=ORIENTED_EDGE('',*,*,#2756,.F.);
#3698=ORIENTED_EDGE('',*,*,#2757,.F.);
#3699=ORIENTED_EDGE('',*,*,#2754,.T.);
#3700=ORIENTED_EDGE('',*,*,#2680,.F.);
#3701=ORIENTED_EDGE('',*,*,#2752,.F.);
#3702=ORIENTED_EDGE('',*,*,#2758,.T.);
#3703=ORIENTED_EDGE('',*,*,#2756,.T.);
#3704=ORIENTED_EDGE('',*,*,#2759,.F.);
#3705=ORIENTED_EDGE('',*,*,#2751,.F.);
#3706=ORIENTED_EDGE('',*,*,#2755,.T.);
#3707=ORIENTED_EDGE('',*,*,#2757,.T.);
#3708=ORIENTED_EDGE('',*,*,#2758,.F.);
#3709=ORIENTED_EDGE('',*,*,#2718,.F.);
#3710=ORIENTED_EDGE('',*,*,#2760,.T.);
#3711=ORIENTED_EDGE('',*,*,#2761,.T.);
#3712=ORIENTED_EDGE('',*,*,#2729,.F.);
#3713=ORIENTED_EDGE('',*,*,#2710,.F.);
#3714=ORIENTED_EDGE('',*,*,#2703,.F.);
#3715=ORIENTED_EDGE('',*,*,#2762,.T.);
#3716=ORIENTED_EDGE('',*,*,#2707,.F.);
#3717=ORIENTED_EDGE('',*,*,#2674,.F.);
#3718=ORIENTED_EDGE('',*,*,#2740,.T.);
#3719=ORIENTED_EDGE('',*,*,#2763,.T.);
#3720=ORIENTED_EDGE('',*,*,#2721,.T.);
#3721=ORIENTED_EDGE('',*,*,#2763,.F.);
#3722=ORIENTED_EDGE('',*,*,#2739,.T.);
#3723=ORIENTED_EDGE('',*,*,#2764,.T.);
#3724=ORIENTED_EDGE('',*,*,#2720,.T.);
#3725=ORIENTED_EDGE('',*,*,#2764,.F.);
#3726=ORIENTED_EDGE('',*,*,#2753,.T.);
#3727=ORIENTED_EDGE('',*,*,#2765,.T.);
#3728=ORIENTED_EDGE('',*,*,#2733,.T.);
#3729=ORIENTED_EDGE('',*,*,#2765,.F.);
#3730=ORIENTED_EDGE('',*,*,#2747,.T.);
#3731=ORIENTED_EDGE('',*,*,#2766,.T.);
#3732=ORIENTED_EDGE('',*,*,#2668,.T.);
#3733=ORIENTED_EDGE('',*,*,#2669,.T.);
#3734=ORIENTED_EDGE('',*,*,#2766,.F.);
#3735=ORIENTED_EDGE('',*,*,#2759,.T.);
#3736=ORIENTED_EDGE('',*,*,#2767,.T.);
#3737=ORIENTED_EDGE('',*,*,#2731,.T.);
#3738=ORIENTED_EDGE('',*,*,#2767,.F.);
#3739=ORIENTED_EDGE('',*,*,#2748,.F.);
#3740=ORIENTED_EDGE('',*,*,#2768,.T.);
#3741=ORIENTED_EDGE('',*,*,#2661,.T.);
#3742=ORIENTED_EDGE('',*,*,#2662,.T.);
#3743=ORIENTED_EDGE('',*,*,#2768,.F.);
#3744=ORIENTED_EDGE('',*,*,#2725,.T.);
#3745=ORIENTED_EDGE('',*,*,#2769,.T.);
#3746=ORIENTED_EDGE('',*,*,#2714,.F.);
#3747=ORIENTED_EDGE('',*,*,#2770,.T.);
#3748=ORIENTED_EDGE('',*,*,#2712,.T.);
#3749=ORIENTED_EDGE('',*,*,#2771,.T.);
#3750=ORIENTED_EDGE('',*,*,#2727,.F.);
#3751=ORIENTED_EDGE('',*,*,#2772,.T.);
#3752=ORIENTED_EDGE('',*,*,#2773,.F.);
#3753=ORIENTED_EDGE('',*,*,#2774,.T.);
#3754=ORIENTED_EDGE('',*,*,#2775,.T.);
#3755=ORIENTED_EDGE('',*,*,#2760,.F.);
#3756=ORIENTED_EDGE('',*,*,#2717,.T.);
#3757=ORIENTED_EDGE('',*,*,#2774,.F.);
#3758=ORIENTED_EDGE('',*,*,#2773,.T.);
#3759=ORIENTED_EDGE('',*,*,#2775,.F.);
#3760=ORIENTED_EDGE('',*,*,#2716,.F.);
#3761=ORIENTED_EDGE('',*,*,#2705,.F.);
#3762=ORIENTED_EDGE('',*,*,#2732,.F.);
#3763=ORIENTED_EDGE('',*,*,#2761,.F.);
#3764=ORIENTED_EDGE('',*,*,#2715,.F.);
#3765=ORIENTED_EDGE('',*,*,#2769,.F.);
#3766=ORIENTED_EDGE('',*,*,#2724,.F.);
#3767=ORIENTED_EDGE('',*,*,#2663,.F.);
#3768=ORIENTED_EDGE('',*,*,#2660,.F.);
#3769=ORIENTED_EDGE('',*,*,#2670,.F.);
#3770=ORIENTED_EDGE('',*,*,#2667,.F.);
#3771=ORIENTED_EDGE('',*,*,#2728,.F.);
#3772=ORIENTED_EDGE('',*,*,#2771,.F.);
#3773=ORIENTED_EDGE('',*,*,#2719,.F.);
#3774=ORIENTED_EDGE('',*,*,#2713,.F.);
#3775=ORIENTED_EDGE('',*,*,#2772,.F.);
#3776=ORIENTED_EDGE('',*,*,#2726,.F.);
#3777=ORIENTED_EDGE('',*,*,#2770,.F.);
#3778=ORIENTED_EDGE('',*,*,#2695,.F.);
#3779=ORIENTED_EDGE('',*,*,#2708,.F.);
#3780=ORIENTED_EDGE('',*,*,#2776,.F.);
#3781=ORIENTED_EDGE('',*,*,#2722,.F.);
#3782=ORIENTED_EDGE('',*,*,#2776,.T.);
#3783=ORIENTED_EDGE('',*,*,#2762,.F.);
#3784=ORIENTED_EDGE('',*,*,#2777,.F.);
#3785=ORIENTED_EDGE('',*,*,#2683,.F.);
#3786=ORIENTED_EDGE('',*,*,#2723,.F.);
#3787=ORIENTED_EDGE('',*,*,#2777,.T.);
#3788=ORIENTED_EDGE('',*,*,#2702,.F.);
#4308=PLANE('',#4883);
#4309=PLANE('',#4886);
#4310=PLANE('',#4889);
#4311=PLANE('',#4891);
#4312=PLANE('',#4893);
#4313=PLANE('',#4894);
#4314=PLANE('',#4896);
#4315=PLANE('',#4898);
#4316=PLANE('',#4900);
#4317=PLANE('',#4907);
#4318=PLANE('',#4911);
#4319=PLANE('',#4913);
#4320=PLANE('',#4915);
#4321=PLANE('',#4918);
#4322=PLANE('',#4919);
#4323=PLANE('',#4920);
#4324=PLANE('',#4922);
#4325=PLANE('',#4924);
#4326=PLANE('',#4925);
#4327=PLANE('',#4926);
#4328=PLANE('',#4928);
#4329=PLANE('',#4929);
#4330=PLANE('',#4930);
#4331=PLANE('',#4932);
#4332=PLANE('',#4943);
#4333=PLANE('',#4944);
#4334=PLANE('',#4947);
#4499=ADVANCED_FACE('',(#558),#4308,.T.);
#4500=ADVANCED_FACE('',(#559),#4309,.F.);
#4501=ADVANCED_FACE('',(#560,#407),#4310,.T.);
#4502=ADVANCED_FACE('',(#561,#408),#4311,.T.);
#4503=ADVANCED_FACE('',(#562),#4312,.T.);
#4504=ADVANCED_FACE('',(#563,#409),#4313,.T.);
#4505=ADVANCED_FACE('',(#564),#4314,.F.);
#4506=ADVANCED_FACE('',(#565),#4315,.F.);
#4507=ADVANCED_FACE('',(#566,#410,#411),#4316,.T.);
#4508=ADVANCED_FACE('',(#567),#4317,.F.);
#4509=ADVANCED_FACE('',(#568,#412),#4318,.T.);
#4510=ADVANCED_FACE('',(#569,#413),#4319,.F.);
#4511=ADVANCED_FACE('',(#570,#414,#415),#4320,.T.);
#4512=ADVANCED_FACE('',(#571),#4321,.F.);
#4513=ADVANCED_FACE('',(#572),#4322,.F.);
#4514=ADVANCED_FACE('',(#573,#416),#4323,.T.);
#4515=ADVANCED_FACE('',(#574,#417),#4324,.F.);
#4516=ADVANCED_FACE('',(#575),#4325,.T.);
#4517=ADVANCED_FACE('',(#576),#4326,.T.);
#4518=ADVANCED_FACE('',(#577,#418),#4327,.T.);
#4519=ADVANCED_FACE('',(#578),#4328,.F.);
#4520=ADVANCED_FACE('',(#579),#4329,.F.);
#4521=ADVANCED_FACE('',(#580,#419),#4330,.T.);
#4522=ADVANCED_FACE('',(#581),#4331,.T.);
#4523=ADVANCED_FACE('',(#582),#224,.F.);
#4524=ADVANCED_FACE('',(#583),#225,.T.);
#4525=ADVANCED_FACE('',(#584),#226,.F.);
#4526=ADVANCED_FACE('',(#585),#227,.F.);
#4527=ADVANCED_FACE('',(#586),#228,.F.);
#4528=ADVANCED_FACE('',(#587),#229,.F.);
#4529=ADVANCED_FACE('',(#588),#230,.F.);
#4530=ADVANCED_FACE('',(#589),#231,.F.);
#4531=ADVANCED_FACE('',(#590),#4332,.T.);
#4532=ADVANCED_FACE('',(#591),#4333,.T.);
#4533=ADVANCED_FACE('',(#592),#232,.F.);
#4534=ADVANCED_FACE('',(#593),#4334,.T.);
#4535=ADVANCED_FACE('',(#594),#233,.F.);
#4536=ADVANCED_FACE('',(#595),#234,.F.);
#4537=ADVANCED_FACE('',(#596),#235,.F.);
#4538=ADVANCED_FACE('',(#597),#236,.T.);
#4539=ADVANCED_FACE('',(#598),#237,.T.);
#4540=ADVANCED_FACE('',(#599),#163,.T.);
#4541=ADVANCED_FACE('',(#600),#238,.T.);
#4632=CLOSED_SHELL('',(#4499,#4500,#4501,#4502,#4503,#4504,#4505,#4506,
#4507,#4508,#4509,#4510,#4511,#4512,#4513,#4514,#4515,#4516,#4517,#4518,
#4519,#4520,#4521,#4522,#4523,#4524,#4525,#4526,#4527,#4528,#4529,#4530,
#4531,#4532,#4533,#4534,#4535,#4536,#4537,#4538,#4539,#4540,#4541));
#4882=AXIS2_PLACEMENT_3D('',#6997,#5671,#5672);
#4883=AXIS2_PLACEMENT_3D('',#6998,#5673,#5674);
#4884=AXIS2_PLACEMENT_3D('',#7005,#5677,#5678);
#4885=AXIS2_PLACEMENT_3D('',#7006,#5679,#5680);
#4886=AXIS2_PLACEMENT_3D('',#7012,#5684,#5685);
#4887=AXIS2_PLACEMENT_3D('',#7019,#5688,#5689);
#4888=AXIS2_PLACEMENT_3D('',#7020,#5690,#5691);
#4889=AXIS2_PLACEMENT_3D('',#7026,#5695,#5696);
#4890=AXIS2_PLACEMENT_3D('',#7031,#5698,#5699);
#4891=AXIS2_PLACEMENT_3D('',#7045,#5707,#5708);
#4892=AXIS2_PLACEMENT_3D('',#7049,#5710,#5711);
#4893=AXIS2_PLACEMENT_3D('',#7061,#5718,#5719);
#4894=AXIS2_PLACEMENT_3D('',#7070,#5724,#5725);
#4895=AXIS2_PLACEMENT_3D('',#7075,#5727,#5728);
#4896=AXIS2_PLACEMENT_3D('',#7086,#5735,#5736);
#4897=AXIS2_PLACEMENT_3D('',#7093,#5740,#5741);
#4898=AXIS2_PLACEMENT_3D('',#7095,#5743,#5744);
#4899=AXIS2_PLACEMENT_3D('',#7102,#5748,#5749);
#4900=AXIS2_PLACEMENT_3D('',#7104,#5751,#5752);
#4901=AXIS2_PLACEMENT_3D('',#7109,#5754,#5755);
#4902=AXIS2_PLACEMENT_3D('',#7112,#5757,#5758);
#4903=AXIS2_PLACEMENT_3D('',#7116,#5760,#5761);
#4904=AXIS2_PLACEMENT_3D('',#7118,#5763,#5764);
#4905=AXIS2_PLACEMENT_3D('',#7120,#5765,#5766);
#4906=AXIS2_PLACEMENT_3D('',#7122,#5767,#5768);
#4907=AXIS2_PLACEMENT_3D('',#7123,#5769,#5770);
#4908=AXIS2_PLACEMENT_3D('',#7128,#5773,#5774);
#4909=AXIS2_PLACEMENT_3D('',#7132,#5776,#5777);
#4910=AXIS2_PLACEMENT_3D('',#7135,#5779,#5780);
#4911=AXIS2_PLACEMENT_3D('',#7136,#5781,#5782);
#4912=AXIS2_PLACEMENT_3D('',#7141,#5785,#5786);
#4913=AXIS2_PLACEMENT_3D('',#7142,#5787,#5788);
#4914=AXIS2_PLACEMENT_3D('',#7145,#5790,#5791);
#4915=AXIS2_PLACEMENT_3D('',#7146,#5792,#5793);
#4916=AXIS2_PLACEMENT_3D('',#7155,#5799,#5800);
#4917=AXIS2_PLACEMENT_3D('',#7157,#5801,#5802);
#4918=AXIS2_PLACEMENT_3D('',#7158,#5803,#5804);
#4919=AXIS2_PLACEMENT_3D('',#7160,#5806,#5807);
#4920=AXIS2_PLACEMENT_3D('',#7167,#5812,#5813);
#4921=AXIS2_PLACEMENT_3D('',#7170,#5815,#5816);
#4922=AXIS2_PLACEMENT_3D('',#7171,#5817,#5818);
#4923=AXIS2_PLACEMENT_3D('',#7173,#5819,#5820);
#4924=AXIS2_PLACEMENT_3D('',#7174,#5821,#5822);
#4925=AXIS2_PLACEMENT_3D('',#7176,#5824,#5825);
#4926=AXIS2_PLACEMENT_3D('',#7177,#5826,#5827);
#4927=AXIS2_PLACEMENT_3D('',#7184,#5831,#5832);
#4928=AXIS2_PLACEMENT_3D('',#7185,#5833,#5834);
#4929=AXIS2_PLACEMENT_3D('',#7189,#5837,#5838);
#4930=AXIS2_PLACEMENT_3D('',#7193,#5841,#5842);
#4931=AXIS2_PLACEMENT_3D('',#7196,#5844,#5845);
#4932=AXIS2_PLACEMENT_3D('',#7197,#5846,#5847);
#4933=AXIS2_PLACEMENT_3D('',#7198,#5848,#5849);
#4934=AXIS2_PLACEMENT_3D('',#7206,#5850,#5851);
#4935=AXIS2_PLACEMENT_3D('',#7207,#5852,#5853);
#4936=AXIS2_PLACEMENT_3D('',#7208,#5854,#5855);
#4937=AXIS2_PLACEMENT_3D('',#7209,#5856,#5857);
#4938=AXIS2_PLACEMENT_3D('',#7211,#5859,#5860);
#4939=AXIS2_PLACEMENT_3D('',#7213,#5862,#5863);
#4940=AXIS2_PLACEMENT_3D('',#7215,#5865,#5866);
#4941=AXIS2_PLACEMENT_3D('',#7217,#5868,#5869);
#4942=AXIS2_PLACEMENT_3D('',#7219,#5871,#5872);
#4943=AXIS2_PLACEMENT_3D('',#7221,#5874,#5875);
#4944=AXIS2_PLACEMENT_3D('',#7224,#5878,#5879);
#4945=AXIS2_PLACEMENT_3D('',#7227,#5882,#5883);
#4946=AXIS2_PLACEMENT_3D('',#7229,#5884,#5885);
#4947=AXIS2_PLACEMENT_3D('',#7237,#5887,#5888);
#4948=AXIS2_PLACEMENT_3D('',#7238,#5889,#5890);
#4949=AXIS2_PLACEMENT_3D('',#7239,#5891,#5892);
#4950=AXIS2_PLACEMENT_3D('',#7240,#5893,#5894);
#4951=AXIS2_PLACEMENT_3D('',#7241,#5895,#5896);
#4952=AXIS2_PLACEMENT_3D('',#7242,#5897,#5898);
#4953=AXIS2_PLACEMENT_3D('',#7243,#5899,#5900);
#4954=AXIS2_PLACEMENT_3D('',#7244,#5901,#5902);
#4955=AXIS2_PLACEMENT_3D('',#7245,#5903,#5904);
#4956=AXIS2_PLACEMENT_3D('',#7246,#5905,#5906);
#5671=DIRECTION('axis',(0.,0.,1.));
#5672=DIRECTION('refdir',(1.,0.,0.));
#5673=DIRECTION('center_axis',(1.,0.,0.));
#5674=DIRECTION('ref_axis',(0.,0.,-1.));
#5675=DIRECTION('',(0.,-1.,0.));
#5676=DIRECTION('',(0.,4.95635278850516E-17,-1.));
#5677=DIRECTION('center_axis',(1.,0.,0.));
#5678=DIRECTION('ref_axis',(0.,0.,-1.));
#5679=DIRECTION('center_axis',(1.,0.,0.));
#5680=DIRECTION('ref_axis',(0.,0.,-1.));
#5681=DIRECTION('',(0.,4.95635278850516E-17,-1.));
#5682=DIRECTION('',(0.,-1.,0.));
#5683=DIRECTION('',(0.,0.,-1.));
#5684=DIRECTION('center_axis',(0.,-1.,0.));
#5685=DIRECTION('ref_axis',(0.,0.,-1.));
#5686=DIRECTION('',(1.,0.,0.));
#5687=DIRECTION('',(0.,0.,-1.));
#5688=DIRECTION('center_axis',(0.,1.,0.));
#5689=DIRECTION('ref_axis',(0.,0.,1.));
#5690=DIRECTION('center_axis',(0.,1.,0.));
#5691=DIRECTION('ref_axis',(0.,0.,1.));
#5692=DIRECTION('',(0.,0.,-1.));
#5693=DIRECTION('',(1.,0.,0.));
#5694=DIRECTION('',(0.,0.,-1.));
#5695=DIRECTION('center_axis',(0.,0.,1.));
#5696=DIRECTION('ref_axis',(1.,0.,0.));
#5697=DIRECTION('',(6.12323399573677E-17,-1.,0.));
#5698=DIRECTION('center_axis',(0.,0.,1.));
#5699=DIRECTION('ref_axis',(1.,0.,0.));
#5700=DIRECTION('',(1.,0.,0.));
#5701=DIRECTION('',(0.,-1.,0.));
#5702=DIRECTION('',(-1.,0.,0.));
#5703=DIRECTION('',(2.00160401074247E-16,-1.,0.));
#5704=DIRECTION('',(1.,0.,0.));
#5705=DIRECTION('',(2.66880534765662E-16,-1.,0.));
#5706=DIRECTION('',(1.,0.,0.));
#5707=DIRECTION('center_axis',(0.,1.,0.));
#5708=DIRECTION('ref_axis',(0.,0.,1.));
#5709=DIRECTION('',(1.,0.,0.));
#5710=DIRECTION('center_axis',(0.,1.,0.));
#5711=DIRECTION('ref_axis',(0.,0.,1.));
#5712=DIRECTION('',(0.,0.,-1.));
#5713=DIRECTION('',(1.,0.,0.));
#5714=DIRECTION('',(0.,0.,-1.));
#5715=DIRECTION('',(-1.,0.,2.66880534765662E-16));
#5716=DIRECTION('',(0.,0.,-1.));
#5717=DIRECTION('',(-1.,0.,2.00160401074247E-16));
#5718=DIRECTION('center_axis',(1.,0.,0.));
#5719=DIRECTION('ref_axis',(0.,1.,0.));
#5720=DIRECTION('',(0.,1.,2.00160401074247E-16));
#5721=DIRECTION('',(0.,0.,1.));
#5722=DIRECTION('',(0.,1.,2.66880534765662E-16));
#5723=DIRECTION('',(0.,0.,-1.));
#5724=DIRECTION('center_axis',(1.,0.,0.));
#5725=DIRECTION('ref_axis',(0.,0.,-1.));
#5726=DIRECTION('',(0.,0.,-1.));
#5727=DIRECTION('center_axis',(1.,0.,0.));
#5728=DIRECTION('ref_axis',(0.,0.,-1.));
#5729=DIRECTION('',(0.,-1.,0.));
#5730=DIRECTION('',(0.,-1.,0.));
#5731=DIRECTION('',(0.,0.,-1.));
#5732=DIRECTION('',(0.,1.,2.66880534765662E-16));
#5733=DIRECTION('',(0.,0.,-1.));
#5734=DIRECTION('',(0.,1.,2.00160401074247E-16));
#5735=DIRECTION('center_axis',(1.,6.12323399573677E-17,0.));
#5736=DIRECTION('ref_axis',(-6.12323399573677E-17,1.,0.));
#5737=DIRECTION('',(6.12323399573677E-17,-1.,0.));
#5738=DIRECTION('',(0.,0.,-1.));
#5739=DIRECTION('',(0.,0.,-1.));
#5740=DIRECTION('center_axis',(1.,6.12323399573677E-17,0.));
#5741=DIRECTION('ref_axis',(-6.12323399573677E-17,1.,0.));
#5742=DIRECTION('',(6.12323399573677E-17,-1.,0.));
#5743=DIRECTION('center_axis',(0.,1.,0.));
#5744=DIRECTION('ref_axis',(0.,0.,1.));
#5745=DIRECTION('',(0.,0.,-1.));
#5746=DIRECTION('',(1.,0.,0.));
#5747=DIRECTION('',(1.,0.,0.));
#5748=DIRECTION('center_axis',(0.,1.,0.));
#5749=DIRECTION('ref_axis',(0.,0.,1.));
#5750=DIRECTION('',(0.,0.,-1.));
#5751=DIRECTION('center_axis',(0.,0.,1.));
#5752=DIRECTION('ref_axis',(1.,0.,0.));
#5753=DIRECTION('',(0.,-1.,0.));
#5754=DIRECTION('center_axis',(0.,0.,1.));
#5755=DIRECTION('ref_axis',(1.,0.,0.));
#5756=DIRECTION('',(-1.,0.,0.));
#5757=DIRECTION('center_axis',(0.,0.,1.));
#5758=DIRECTION('ref_axis',(1.,0.,0.));
#5759=DIRECTION('',(-1.,0.,0.));
#5760=DIRECTION('center_axis',(0.,0.,1.));
#5761=DIRECTION('ref_axis',(1.,0.,0.));
#5762=DIRECTION('',(0.,-1.,0.));
#5763=DIRECTION('center_axis',(0.,0.,1.));
#5764=DIRECTION('ref_axis',(1.,0.,0.));
#5765=DIRECTION('center_axis',(0.,0.,1.));
#5766=DIRECTION('ref_axis',(1.,0.,0.));
#5767=DIRECTION('center_axis',(0.,0.,1.));
#5768=DIRECTION('ref_axis',(1.,0.,0.));
#5769=DIRECTION('center_axis',(0.,0.,1.));
#5770=DIRECTION('ref_axis',(1.,0.,0.));
#5771=DIRECTION('',(1.,0.,0.));
#5772=DIRECTION('',(6.12323399573677E-17,-1.,0.));
#5773=DIRECTION('center_axis',(0.,0.,1.));
#5774=DIRECTION('ref_axis',(1.,0.,0.));
#5775=DIRECTION('',(-1.,0.,0.));
#5776=DIRECTION('center_axis',(0.,0.,1.));
#5777=DIRECTION('ref_axis',(1.,0.,0.));
#5778=DIRECTION('',(0.,-1.,0.));
#5779=DIRECTION('center_axis',(0.,0.,1.));
#5780=DIRECTION('ref_axis',(1.,0.,0.));
#5781=DIRECTION('center_axis',(1.,0.,0.));
#5782=DIRECTION('ref_axis',(0.,0.,-1.));
#5783=DIRECTION('',(0.,-1.,0.));
#5784=DIRECTION('',(0.,0.,-1.));
#5785=DIRECTION('center_axis',(1.,0.,0.));
#5786=DIRECTION('ref_axis',(0.,0.,-1.));
#5787=DIRECTION('center_axis',(0.,-1.,0.));
#5788=DIRECTION('ref_axis',(0.,0.,-1.));
#5789=DIRECTION('',(-1.,0.,0.));
#5790=DIRECTION('center_axis',(0.,1.,0.));
#5791=DIRECTION('ref_axis',(0.,0.,1.));
#5792=DIRECTION('center_axis',(0.,2.66880534765662E-16,-1.));
#5793=DIRECTION('ref_axis',(0.,1.,2.66880534765662E-16));
#5794=DIRECTION('',(-1.,0.,2.66880534765662E-16));
#5795=DIRECTION('',(0.,1.,0.));
#5796=DIRECTION('',(0.,1.,0.));
#5797=DIRECTION('',(1.,0.,0.));
#5798=DIRECTION('',(1.,0.,0.));
#5799=DIRECTION('center_axis',(0.,2.66880534765662E-16,-1.));
#5800=DIRECTION('ref_axis',(0.,1.,2.66880534765662E-16));
#5801=DIRECTION('center_axis',(0.,2.66880534765662E-16,-1.));
#5802=DIRECTION('ref_axis',(0.,1.,2.66880534765662E-16));
#5803=DIRECTION('center_axis',(0.,-1.,0.));
#5804=DIRECTION('ref_axis',(0.,0.,-1.));
#5805=DIRECTION('',(1.,0.,0.));
#5806=DIRECTION('center_axis',(0.,2.00160401074247E-16,-1.));
#5807=DIRECTION('ref_axis',(0.,1.,2.00160401074247E-16));
#5808=DIRECTION('',(1.,0.,0.));
#5809=DIRECTION('',(0.,1.,0.));
#5810=DIRECTION('',(0.,1.,0.));
#5811=DIRECTION('',(-1.,0.,2.00160401074247E-16));
#5812=DIRECTION('center_axis',(0.,-1.,0.));
#5813=DIRECTION('ref_axis',(0.,0.,-1.));
#5814=DIRECTION('',(0.,0.,1.));
#5815=DIRECTION('center_axis',(0.,-1.,0.));
#5816=DIRECTION('ref_axis',(0.,0.,-1.));
#5817=DIRECTION('center_axis',(1.,0.,0.));
#5818=DIRECTION('ref_axis',(0.,0.,-1.));
#5819=DIRECTION('center_axis',(1.,0.,0.));
#5820=DIRECTION('ref_axis',(0.,0.,-1.));
#5821=DIRECTION('center_axis',(1.,0.,0.));
#5822=DIRECTION('ref_axis',(0.,0.,-1.));
#5823=DIRECTION('',(0.,0.,-1.));
#5824=DIRECTION('center_axis',(0.,1.,0.));
#5825=DIRECTION('ref_axis',(-1.,0.,0.));
#5826=DIRECTION('center_axis',(0.,-1.,0.));
#5827=DIRECTION('ref_axis',(0.,0.,-1.));
#5828=DIRECTION('',(0.,0.,1.));
#5829=DIRECTION('',(1.,0.,0.));
#5830=DIRECTION('',(0.,0.,1.));
#5831=DIRECTION('center_axis',(0.,-1.,0.));
#5832=DIRECTION('ref_axis',(0.,0.,-1.));
#5833=DIRECTION('center_axis',(-1.,-2.00160401074247E-16,0.));
#5834=DIRECTION('ref_axis',(2.00160401074247E-16,-1.,0.));
#5835=DIRECTION('',(0.,0.,1.));
#5836=DIRECTION('',(2.00160401074247E-16,-1.,0.));
#5837=DIRECTION('center_axis',(0.,-1.,0.));
#5838=DIRECTION('ref_axis',(0.,0.,-1.));
#5839=DIRECTION('',(0.,0.,1.));
#5840=DIRECTION('',(1.,0.,0.));
#5841=DIRECTION('center_axis',(-1.,-2.66880534765662E-16,0.));
#5842=DIRECTION('ref_axis',(2.66880534765662E-16,-1.,0.));
#5843=DIRECTION('',(2.66880534765662E-16,-1.,0.));
#5844=DIRECTION('center_axis',(-1.,-2.66880534765662E-16,0.));
#5845=DIRECTION('ref_axis',(2.66880534765662E-16,-1.,0.));
#5846=DIRECTION('center_axis',(0.,0.,1.));
#5847=DIRECTION('ref_axis',(1.,0.,0.));
#5848=DIRECTION('center_axis',(0.,1.,0.));
#5849=DIRECTION('ref_axis',(0.,0.,1.));
#5850=DIRECTION('center_axis',(-0.707106781186548,0.707106781186548,0.));
#5851=DIRECTION('ref_axis',(0.707106781186547,0.707106781186547,0.));
#5852=DIRECTION('center_axis',(0.,0.,-1.));
#5853=DIRECTION('ref_axis',(-1.,0.,0.));
#5854=DIRECTION('center_axis',(0.,0.,-1.));
#5855=DIRECTION('ref_axis',(-1.,0.,0.));
#5856=DIRECTION('center_axis',(0.,0.,1.));
#5857=DIRECTION('ref_axis',(1.,0.,0.));
#5858=DIRECTION('',(0.,0.,1.));
#5859=DIRECTION('center_axis',(0.,0.,1.));
#5860=DIRECTION('ref_axis',(1.,0.,0.));
#5861=DIRECTION('',(0.,0.,1.));
#5862=DIRECTION('center_axis',(0.,1.,0.));
#5863=DIRECTION('ref_axis',(0.,0.,1.));
#5864=DIRECTION('',(0.,1.,0.));
#5865=DIRECTION('center_axis',(0.,1.,0.));
#5866=DIRECTION('ref_axis',(0.,0.,1.));
#5867=DIRECTION('',(0.,1.,0.));
#5868=DIRECTION('center_axis',(1.,0.,0.));
#5869=DIRECTION('ref_axis',(0.,0.,-1.));
#5870=DIRECTION('',(1.,0.,0.));
#5871=DIRECTION('center_axis',(1.,0.,0.));
#5872=DIRECTION('ref_axis',(0.,0.,-1.));
#5873=DIRECTION('',(1.,0.,0.));
#5874=DIRECTION('center_axis',(0.,1.,4.95635278850516E-17));
#5875=DIRECTION('ref_axis',(0.,-4.95635278850516E-17,1.));
#5876=DIRECTION('',(0.,4.95635278850516E-17,-1.));
#5877=DIRECTION('',(0.,4.95635278850516E-17,-1.));
#5878=DIRECTION('center_axis',(1.,0.,0.));
#5879=DIRECTION('ref_axis',(0.,1.,0.));
#5880=DIRECTION('',(0.,0.,-1.));
#5881=DIRECTION('',(0.,4.95635278850516E-17,-1.));
#5882=DIRECTION('center_axis',(0.,0.,1.));
#5883=DIRECTION('ref_axis',(1.,0.,0.));
#5884=DIRECTION('center_axis',(0.,0.,1.));
#5885=DIRECTION('ref_axis',(1.,0.,0.));
#5886=DIRECTION('',(0.,0.,1.));
#5887=DIRECTION('center_axis',(0.,0.,1.));
#5888=DIRECTION('ref_axis',(1.,0.,0.));
#5889=DIRECTION('center_axis',(-1.,0.,0.));
#5890=DIRECTION('ref_axis',(0.,0.,1.));
#5891=DIRECTION('center_axis',(0.,-4.95635278850516E-17,1.));
#5892=DIRECTION('ref_axis',(0.,-1.,-4.95635278850516E-17));
#5893=DIRECTION('center_axis',(0.,0.,-1.));
#5894=DIRECTION('ref_axis',(-1.,0.,0.));
#5895=DIRECTION('center_axis',(0.,4.95635278850516E-17,-1.));
#5896=DIRECTION('ref_axis',(0.,1.,4.95635278850516E-17));
#5897=DIRECTION('center_axis',(1.,0.,0.));
#5898=DIRECTION('ref_axis',(0.,0.,-1.));
#5899=DIRECTION('center_axis',(-1.,0.,0.));
#5900=DIRECTION('ref_axis',(0.,0.,1.));
#5901=DIRECTION('center_axis',(0.,0.,1.));
#5902=DIRECTION('ref_axis',(1.,0.,0.));
#5903=DIRECTION('center_axis',(0.,1.,0.));
#5904=DIRECTION('ref_axis',(0.,0.,1.));
#5905=DIRECTION('center_axis',(6.12323399573677E-17,-1.,0.));
#5906=DIRECTION('ref_axis',(1.,6.12323399573677E-17,0.));
#6997=CARTESIAN_POINT('',(0.,0.,0.));
#6998=CARTESIAN_POINT('Origin',(0.035,0.002224231518171,0.035));
#6999=CARTESIAN_POINT('',(0.035,0.032224231518171,0.035));
#7000=CARTESIAN_POINT('',(0.035,0.012224231518171,0.035));
#7001=CARTESIAN_POINT('',(0.035,0.002224231518171,0.035));
#7002=CARTESIAN_POINT('',(0.035,0.012224231518171,0.0175));
#7003=CARTESIAN_POINT('',(0.035,0.012224231518171,0.));
#7004=CARTESIAN_POINT('',(0.035,0.014724231518171,0.02));
#7005=CARTESIAN_POINT('Origin',(0.035,0.014724231518171,0.0175));
#7006=CARTESIAN_POINT('Origin',(0.035,0.014724231518171,0.0175));
#7007=CARTESIAN_POINT('',(0.035,0.012224231518171,0.));
#7008=CARTESIAN_POINT('',(0.035,0.012224231518171,0.));
#7009=CARTESIAN_POINT('',(0.035,0.032224231518171,0.));
#7010=CARTESIAN_POINT('',(0.035,0.002224231518171,0.));
#7011=CARTESIAN_POINT('',(0.035,0.032224231518171,0.035));
#7012=CARTESIAN_POINT('Origin',(0.0175,-0.027775768481829,0.095));
#7013=CARTESIAN_POINT('',(0.075,-0.027775768481829,0.));
#7014=CARTESIAN_POINT('',(0.095,-0.027775768481829,0.));
#7015=CARTESIAN_POINT('',(0.065,-0.027775768481829,0.));
#7016=CARTESIAN_POINT('',(0.075,-0.027775768481829,0.0175));
#7017=CARTESIAN_POINT('',(0.075,-0.027775768481829,0.095));
#7018=CARTESIAN_POINT('',(0.0775,-0.027775768481829,0.015));
#7019=CARTESIAN_POINT('Origin',(0.0775,-0.027775768481829,0.0175));
#7020=CARTESIAN_POINT('Origin',(0.0775,-0.027775768481829,0.0175));
#7021=CARTESIAN_POINT('',(0.075,-0.027775768481829,0.035));
#7022=CARTESIAN_POINT('',(0.075,-0.027775768481829,0.095));
#7023=CARTESIAN_POINT('',(0.095,-0.027775768481829,0.035));
#7024=CARTESIAN_POINT('',(0.065,-0.027775768481829,0.035));
#7025=CARTESIAN_POINT('',(0.095,-0.027775768481829,0.035));
#7026=CARTESIAN_POINT('Origin',(0.0475,-0.015275768481829,0.095));
#7027=CARTESIAN_POINT('',(1.81423519728374E-18,-0.027775768481829,0.095));
#7028=CARTESIAN_POINT('',(3.2225790163032E-18,-0.050775768481829,0.095));
#7029=CARTESIAN_POINT('',(1.04883094781665E-18,-0.015275768481829,0.095));
#7030=CARTESIAN_POINT('',(0.012,-0.062775768481829,0.095));
#7031=CARTESIAN_POINT('Origin',(0.012,-0.050775768481829,0.095));
#7032=CARTESIAN_POINT('',(0.035,-0.062775768481829,0.095));
#7033=CARTESIAN_POINT('',(0.0475,-0.062775768481829,0.095));
#7034=CARTESIAN_POINT('',(0.035,-0.027775768481829,0.095));
#7035=CARTESIAN_POINT('',(0.035,-0.045275768481829,0.095));
#7036=CARTESIAN_POINT('',(0.0175,-0.027775768481829,0.095));
#7037=CARTESIAN_POINT('',(0.0045,-0.032275768481829,0.095));
#7038=CARTESIAN_POINT('',(0.0045,-0.058275768481829,0.095));
#7039=CARTESIAN_POINT('',(0.0045,-0.045275768481829,0.095));
#7040=CARTESIAN_POINT('',(0.0305,-0.032275768481829,0.095));
#7041=CARTESIAN_POINT('',(0.0175,-0.032275768481829,0.095));
#7042=CARTESIAN_POINT('',(0.0305,-0.058275768481829,0.095));
#7043=CARTESIAN_POINT('',(0.0305,-0.045275768481829,0.095));
#7044=CARTESIAN_POINT('',(0.0175,-0.058275768481829,0.095));
#7045=CARTESIAN_POINT('Origin',(0.0175,0.032224231518171,0.035));
#7046=CARTESIAN_POINT('',(0.012,0.032224231518171,0.));
#7047=CARTESIAN_POINT('',(0.0175,0.032224231518171,0.));
#7048=CARTESIAN_POINT('',(-3.46944695195361E-18,0.032224231518171,0.012));
#7049=CARTESIAN_POINT('Origin',(0.012,0.032224231518171,0.012));
#7050=CARTESIAN_POINT('',(-3.46944695195361E-18,0.032224231518171,0.035));
#7051=CARTESIAN_POINT('',(-3.46944695195361E-18,0.032224231518171,0.035));
#7052=CARTESIAN_POINT('',(0.0175,0.032224231518171,0.035));
#7053=CARTESIAN_POINT('',(0.0305,0.032224231518171,0.0305));
#7054=CARTESIAN_POINT('',(0.0305,0.032224231518171,0.0045));
#7055=CARTESIAN_POINT('',(0.0305,0.032224231518171,0.0175));
#7056=CARTESIAN_POINT('',(0.0045,0.032224231518171,0.0305));
#7057=CARTESIAN_POINT('',(0.0175,0.032224231518171,0.0305));
#7058=CARTESIAN_POINT('',(0.0045,0.032224231518171,0.0045));
#7059=CARTESIAN_POINT('',(0.0045,0.032224231518171,0.0175));
#7060=CARTESIAN_POINT('',(0.0175,0.032224231518171,0.0045));
#7061=CARTESIAN_POINT('Origin',(0.03,-0.045275768481829,0.0175));
#7062=CARTESIAN_POINT('',(0.03,-0.058275768481829,0.0045));
#7063=CARTESIAN_POINT('',(0.03,-0.032775768481829,0.0045));
#7064=CARTESIAN_POINT('',(0.03,-0.045275768481829,0.0045));
#7065=CARTESIAN_POINT('',(0.03,-0.032775768481829,0.0305));
#7066=CARTESIAN_POINT('',(0.03,-0.032775768481829,0.0175));
#7067=CARTESIAN_POINT('',(0.03,-0.058275768481829,0.0305));
#7068=CARTESIAN_POINT('',(0.03,-0.045275768481829,0.0305));
#7069=CARTESIAN_POINT('',(0.03,-0.058275768481829,0.0175));
#7070=CARTESIAN_POINT('Origin',(0.095,-0.045275768481829,0.035));
#7071=CARTESIAN_POINT('',(0.095,-0.062775768481829,0.035));
#7072=CARTESIAN_POINT('',(0.095,-0.062775768481829,0.012));
#7073=CARTESIAN_POINT('',(0.095,-0.062775768481829,0.035));
#7074=CARTESIAN_POINT('',(0.095,-0.050775768481829,0.));
#7075=CARTESIAN_POINT('Origin',(0.095,-0.050775768481829,0.012));
#7076=CARTESIAN_POINT('',(0.095,-0.045275768481829,0.));
#7077=CARTESIAN_POINT('',(0.095,-0.045275768481829,0.035));
#7078=CARTESIAN_POINT('',(0.095,-0.058275768481829,0.0305));
#7079=CARTESIAN_POINT('',(0.095,-0.058275768481829,0.0045));
#7080=CARTESIAN_POINT('',(0.095,-0.058275768481829,0.0175));
#7081=CARTESIAN_POINT('',(0.095,-0.032275768481829,0.0305));
#7082=CARTESIAN_POINT('',(0.095,-0.045275768481829,0.0305));
#7083=CARTESIAN_POINT('',(0.095,-0.032275768481829,0.0045));
#7084=CARTESIAN_POINT('',(0.095,-0.032275768481829,0.0175));
#7085=CARTESIAN_POINT('',(0.095,-0.045275768481829,0.0045));
#7086=CARTESIAN_POINT('Origin',(1.04883094781665E-18,-0.015275768481829,
0.035));
#7087=CARTESIAN_POINT('',(3.2225790163032E-18,-0.050775768481829,0.012));
#7088=CARTESIAN_POINT('',(1.04883094781665E-18,-0.015275768481829,0.012));
#7089=CARTESIAN_POINT('',(3.2225790163032E-18,-0.050775768481829,0.035));
#7090=CARTESIAN_POINT('',(1.81423519728374E-18,-0.027775768481829,0.045));
#7091=CARTESIAN_POINT('',(1.81423519728374E-18,-0.027775768481829,0.095));
#7092=CARTESIAN_POINT('',(1.20191179771007E-18,-0.017775768481829,0.035));
#7093=CARTESIAN_POINT('Origin',(0.,-0.017775768481829,0.045));
#7094=CARTESIAN_POINT('',(1.04883094781665E-18,-0.015275768481829,0.035));
#7095=CARTESIAN_POINT('Origin',(0.0475,-0.062775768481829,0.035));
#7096=CARTESIAN_POINT('',(0.012,-0.062775768481829,0.012));
#7097=CARTESIAN_POINT('',(0.012,-0.062775768481829,0.035));
#7098=CARTESIAN_POINT('',(0.0475,-0.062775768481829,0.012));
#7099=CARTESIAN_POINT('',(0.045,-0.062775768481829,0.035));
#7100=CARTESIAN_POINT('',(0.0475,-0.062775768481829,0.035));
#7101=CARTESIAN_POINT('',(0.035,-0.062775768481829,0.045));
#7102=CARTESIAN_POINT('Origin',(0.045,-0.062775768481829,0.045));
#7103=CARTESIAN_POINT('',(0.035,-0.062775768481829,0.095));
#7104=CARTESIAN_POINT('Origin',(0.0475,-0.015275768481829,0.035));
#7105=CARTESIAN_POINT('',(0.07,0.00222423151817101,0.035));
#7106=CARTESIAN_POINT('',(0.07,-0.022775768481829,0.035));
#7107=CARTESIAN_POINT('',(0.07,0.002224231518171,0.035));
#7108=CARTESIAN_POINT('',(0.065,0.00722423151817101,0.035));
#7109=CARTESIAN_POINT('Origin',(0.065,0.00222423151817101,0.035));
#7110=CARTESIAN_POINT('',(0.04,0.00722423151817101,0.035));
#7111=CARTESIAN_POINT('',(0.07,0.00722423151817101,0.035));
#7112=CARTESIAN_POINT('Origin',(0.04,0.012224231518171,0.035));
#7113=CARTESIAN_POINT('',(0.04075,-0.017775768481829,0.035));
#7114=CARTESIAN_POINT('',(0.0475,-0.017775768481829,0.035));
#7115=CARTESIAN_POINT('',(0.045,-0.022025768481829,0.035));
#7116=CARTESIAN_POINT('Origin',(0.045,-0.017775768481829,0.035));
#7117=CARTESIAN_POINT('',(0.045,-0.062775768481829,0.035));
#7118=CARTESIAN_POINT('Origin',(0.075,-0.022775768481829,0.035));
#7119=CARTESIAN_POINT('',(0.015,0.014724231518171,0.035));
#7120=CARTESIAN_POINT('Origin',(0.0175,0.014724231518171,0.035));
#7121=CARTESIAN_POINT('',(0.075,-0.045275768481829,0.035));
#7122=CARTESIAN_POINT('Origin',(0.0775,-0.045275768481829,0.035));
#7123=CARTESIAN_POINT('Origin',(0.0475,-0.015275768481829,0.));
#7124=CARTESIAN_POINT('',(0.012,-0.050775768481829,0.));
#7125=CARTESIAN_POINT('',(0.0475,-0.050775768481829,0.));
#7126=CARTESIAN_POINT('',(0.012,-0.015275768481829,0.));
#7127=CARTESIAN_POINT('',(0.04,0.00722423151817101,0.));
#7128=CARTESIAN_POINT('Origin',(0.04,0.012224231518171,0.));
#7129=CARTESIAN_POINT('',(0.065,0.00722423151817101,0.));
#7130=CARTESIAN_POINT('',(0.07,0.00722423151817101,0.));
#7131=CARTESIAN_POINT('',(0.07,0.00222423151817101,0.));
#7132=CARTESIAN_POINT('Origin',(0.065,0.00222423151817101,0.));
#7133=CARTESIAN_POINT('',(0.07,-0.022775768481829,0.));
#7134=CARTESIAN_POINT('',(0.07,0.002224231518171,0.));
#7135=CARTESIAN_POINT('Origin',(0.075,-0.022775768481829,0.));
#7136=CARTESIAN_POINT('Origin',(0.035,-0.045275768481829,0.095));
#7137=CARTESIAN_POINT('',(0.035,-0.027775768481829,0.045));
#7138=CARTESIAN_POINT('',(0.035,-0.027775768481829,0.045));
#7139=CARTESIAN_POINT('',(0.035,-0.027775768481829,0.095));
#7140=CARTESIAN_POINT('',(0.035,-0.045275768481829,0.08));
#7141=CARTESIAN_POINT('Origin',(0.035,-0.045275768481829,0.0775));
#7142=CARTESIAN_POINT('Origin',(0.0175,-0.027775768481829,0.095));
#7143=CARTESIAN_POINT('',(0.0175,-0.027775768481829,0.045));
#7144=CARTESIAN_POINT('',(0.0175,-0.027775768481829,0.075));
#7145=CARTESIAN_POINT('Origin',(0.0175,-0.027775768481829,0.0775));
#7146=CARTESIAN_POINT('Origin',(0.03,-0.045275768481829,0.0305));
#7147=CARTESIAN_POINT('',(0.0045,-0.032775768481829,0.0305));
#7148=CARTESIAN_POINT('',(0.0175,-0.032775768481829,0.0305));
#7149=CARTESIAN_POINT('',(0.0045,-0.032775768481829,0.0305));
#7150=CARTESIAN_POINT('',(0.0305,-0.032275768481829,0.0305));
#7151=CARTESIAN_POINT('',(0.0305,-0.032775768481829,0.0305));
#7152=CARTESIAN_POINT('',(0.03,-0.032275768481829,0.0305));
#7153=CARTESIAN_POINT('',(0.03,-0.058275768481829,0.0305));
#7154=CARTESIAN_POINT('',(0.015,0.014724231518171,0.0305));
#7155=CARTESIAN_POINT('Origin',(0.0175,0.014724231518171,0.0305));
#7156=CARTESIAN_POINT('',(0.075,-0.045275768481829,0.0305));
#7157=CARTESIAN_POINT('Origin',(0.0775,-0.045275768481829,0.0305));
#7158=CARTESIAN_POINT('Origin',(0.03,-0.058275768481829,0.0175));
#7159=CARTESIAN_POINT('',(0.03,-0.058275768481829,0.0045));
#7160=CARTESIAN_POINT('Origin',(0.03,-0.045275768481829,0.0045));
#7161=CARTESIAN_POINT('',(0.0305,-0.032275768481829,0.0045));
#7162=CARTESIAN_POINT('',(0.03,-0.032275768481829,0.0045));
#7163=CARTESIAN_POINT('',(0.0305,-0.032775768481829,0.0045));
#7164=CARTESIAN_POINT('',(0.0045,-0.032775768481829,0.0045));
#7165=CARTESIAN_POINT('',(0.0045,-0.032775768481829,0.0045));
#7166=CARTESIAN_POINT('',(0.0175,-0.032775768481829,0.0045));
#7167=CARTESIAN_POINT('Origin',(0.03,-0.032275768481829,0.0175));
#7168=CARTESIAN_POINT('',(0.0305,-0.032275768481829,0.0175));
#7169=CARTESIAN_POINT('',(0.0775,-0.032275768481829,0.015));
#7170=CARTESIAN_POINT('Origin',(0.0775,-0.032275768481829,0.0175));
#7171=CARTESIAN_POINT('Origin',(0.0305,-0.032775768481829,0.0175));
#7172=CARTESIAN_POINT('',(0.0305,0.014724231518171,0.02));
#7173=CARTESIAN_POINT('Origin',(0.0305,0.014724231518171,0.0175));
#7174=CARTESIAN_POINT('Origin',(0.0045,-0.032775768481829,0.0175));
#7175=CARTESIAN_POINT('',(0.0045,-0.032775768481829,0.0175));
#7176=CARTESIAN_POINT('Origin',(0.0175,-0.032775768481829,0.0175));
#7177=CARTESIAN_POINT('Origin',(0.0175,-0.032275768481829,0.035));
#7178=CARTESIAN_POINT('',(0.0045,-0.032275768481829,0.035));
#7179=CARTESIAN_POINT('',(0.0045,-0.032275768481829,0.035));
#7180=CARTESIAN_POINT('',(0.0305,-0.032275768481829,0.035));
#7181=CARTESIAN_POINT('',(0.0175,-0.032275768481829,0.035));
#7182=CARTESIAN_POINT('',(0.0305,-0.032275768481829,0.035));
#7183=CARTESIAN_POINT('',(0.0175,-0.032275768481829,0.075));
#7184=CARTESIAN_POINT('Origin',(0.0175,-0.032275768481829,0.0775));
#7185=CARTESIAN_POINT('Origin',(0.0045,-0.045275768481829,0.035));
#7186=CARTESIAN_POINT('',(0.0045,-0.058275768481829,0.035));
#7187=CARTESIAN_POINT('',(0.0045,-0.058275768481829,0.035));
#7188=CARTESIAN_POINT('',(0.0045,-0.045275768481829,0.035));
#7189=CARTESIAN_POINT('Origin',(0.0175,-0.058275768481829,0.035));
#7190=CARTESIAN_POINT('',(0.0305,-0.058275768481829,0.035));
#7191=CARTESIAN_POINT('',(0.0305,-0.058275768481829,0.035));
#7192=CARTESIAN_POINT('',(0.0175,-0.058275768481829,0.035));
#7193=CARTESIAN_POINT('Origin',(0.0305,-0.045275768481829,0.035));
#7194=CARTESIAN_POINT('',(0.0305,-0.045275768481829,0.035));
#7195=CARTESIAN_POINT('',(0.0305,-0.045275768481829,0.08));
#7196=CARTESIAN_POINT('Origin',(0.0305,-0.045275768481829,0.0775));
#7197=CARTESIAN_POINT('Origin',(0.0175,-0.045275768481829,0.035));
#7198=CARTESIAN_POINT('Origin',(0.045,-0.015275768481829,0.045));
#7199=CARTESIAN_POINT('',(0.0419947961799572,-0.0207809723018718,0.0354622460715324));
#7200=CARTESIAN_POINT('Ctrl Pts',(0.0419947961799572,-0.0207809723018718,
0.0354622460715324));
#7201=CARTESIAN_POINT('Ctrl Pts',(0.0423680832260346,-0.0211542593479493,
0.0353446288982169));
#7202=CARTESIAN_POINT('Ctrl Pts',(0.0428414808162073,-0.0214803550845837,
0.0352213771897135));
#7203=CARTESIAN_POINT('Ctrl Pts',(0.0438867716250497,-0.0219162865891378,
0.0350480458316003));
#7204=CARTESIAN_POINT('Ctrl Pts',(0.0444591485998935,-0.022025768481829,
0.035));
#7205=CARTESIAN_POINT('Ctrl Pts',(0.045,-0.022025768481829,0.035));
#7206=CARTESIAN_POINT('Origin',(0.045,-0.017775768481829,0.045));
#7207=CARTESIAN_POINT('Origin',(0.012,-0.050775768481829,0.035));
#7208=CARTESIAN_POINT('Origin',(0.012,-0.050775768481829,0.012));
#7209=CARTESIAN_POINT('Origin',(0.0775,-0.045275768481829,0.025));
#7210=CARTESIAN_POINT('',(0.075,-0.045275768481829,0.025));
#7211=CARTESIAN_POINT('Origin',(0.0175,0.014724231518171,0.025));
#7212=CARTESIAN_POINT('',(0.015,0.014724231518171,0.025));
#7213=CARTESIAN_POINT('Origin',(0.0175,-0.037775768481829,0.0775));
#7214=CARTESIAN_POINT('',(0.0175,-0.037775768481829,0.075));
#7215=CARTESIAN_POINT('Origin',(0.0775,-0.037775768481829,0.0175));
#7216=CARTESIAN_POINT('',(0.0775,-0.037775768481829,0.015));
#7217=CARTESIAN_POINT('Origin',(0.025,-0.045275768481829,0.0775));
#7218=CARTESIAN_POINT('',(0.025,-0.045275768481829,0.08));
#7219=CARTESIAN_POINT('Origin',(0.025,0.014724231518171,0.0175));
#7220=CARTESIAN_POINT('',(0.025,0.014724231518171,0.02));
#7221=CARTESIAN_POINT('Origin',(0.07,0.00722423151817101,0.0175));
#7222=CARTESIAN_POINT('',(0.04,0.00722423151817101,0.035));
#7223=CARTESIAN_POINT('',(0.065,0.00722423151817101,0.0175));
#7224=CARTESIAN_POINT('Origin',(0.07,0.002224231518171,0.0175));
#7225=CARTESIAN_POINT('',(0.07,-0.022775768481829,0.0175));
#7226=CARTESIAN_POINT('',(0.07,0.002224231518171,0.0175));
#7227=CARTESIAN_POINT('Origin',(0.045,-0.017775768481829,0.01));
#7228=CARTESIAN_POINT('',(0.04075,-0.017775768481829,0.01));
#7229=CARTESIAN_POINT('Origin',(0.045,-0.017775768481829,0.01));
#7230=CARTESIAN_POINT('',(0.04075,-0.017775768481829,0.01));
#7231=CARTESIAN_POINT('Ctrl Pts',(0.04075,-0.017775768481829,0.035));
#7232=CARTESIAN_POINT('Ctrl Pts',(0.04075,-0.0183166198819355,0.035));
#7233=CARTESIAN_POINT('Ctrl Pts',(0.0408594818926913,-0.0188889968567793,
0.0350480458316003));
#7234=CARTESIAN_POINT('Ctrl Pts',(0.0412954133972453,-0.0199342876656216,
0.0352213771897135));
#7235=CARTESIAN_POINT('Ctrl Pts',(0.0416215091338797,-0.0204076852557944,
0.0353446288982169));
#7236=CARTESIAN_POINT('Ctrl Pts',(0.0419947961799572,-0.0207809723018718,
0.0354622460715324));
#7237=CARTESIAN_POINT('Origin',(0.0475,-0.015275768481829,0.01));
#7238=CARTESIAN_POINT('Origin',(0.0175,-0.017775768481829,0.045));
#7239=CARTESIAN_POINT('Origin',(0.04,0.012224231518171,0.035));
#7240=CARTESIAN_POINT('Origin',(0.075,-0.022775768481829,0.0175));
#7241=CARTESIAN_POINT('Origin',(0.065,0.00222423151817101,0.0175));
#7242=CARTESIAN_POINT('Origin',(0.0475,-0.050775768481829,0.012));
#7243=CARTESIAN_POINT('Origin',(0.012,-0.050775768481829,0.012));
#7244=CARTESIAN_POINT('Origin',(0.012,-0.050775768481829,0.012));
#7245=CARTESIAN_POINT('Origin',(0.012,-0.050775768481829,0.012));
#7246=CARTESIAN_POINT('Origin',(0.012,-0.015275768481829,0.012));
#7742=UNCERTAINTY_MEASURE_WITH_UNIT(LENGTH_MEASURE(1.E-5),#7757,
'DISTANCE_ACCURACY_VALUE',
'Maximum model space distance between geometric entities at asserted c
onnectivities');
#7745=UNCERTAINTY_MEASURE_WITH_UNIT(LENGTH_MEASURE(1.E-5),#7757,
'DISTANCE_ACCURACY_VALUE',
'Maximum model space distance between geometric entities at asserted c
onnectivities');
#7753=(
GEOMETRIC_REPRESENTATION_CONTEXT(3)
GLOBAL_UNCERTAINTY_ASSIGNED_CONTEXT((#7742))
GLOBAL_UNIT_ASSIGNED_CONTEXT((#7757,#7758,#7759))
REPRESENTATION_CONTEXT('','3D')
);
#7756=(
GEOMETRIC_REPRESENTATION_CONTEXT(3)
GLOBAL_UNCERTAINTY_ASSIGNED_CONTEXT((#7745))
GLOBAL_UNIT_ASSIGNED_CONTEXT((#7757,#7758,#7759))
REPRESENTATION_CONTEXT('','3D')
);
#7757=(
LENGTH_UNIT()
NAMED_UNIT(*)
SI_UNIT($,.METRE.)
);
#7758=(
NAMED_UNIT(*)
PLANE_ANGLE_UNIT()
SI_UNIT($,.RADIAN.)
);
#7759=(
NAMED_UNIT(*)
SI_UNIT($,.STERADIAN.)
SOLID_ANGLE_UNIT()
);
#7767=SHAPE_DEFINITION_REPRESENTATION(#7777,#7825);
#7777=PRODUCT_DEFINITION_SHAPE('',$,#7836);
#7825=SHAPE_REPRESENTATION('',(#4882),#7753);
#7828=PRODUCT_DEFINITION_CONTEXT('part definition',#7860,'design');
#7836=PRODUCT_DEFINITION('Corner Bracket','Corner Bracket',#7846,#7828);
#7846=PRODUCT_DEFINITION_FORMATION('',$,#7869);
#7860=APPLICATION_CONTEXT(
'Core Data for Automotive Mechanical Design Process');
#7861=PRODUCT_CONTEXT('part definition',#7860,'mechanical');
#7869=PRODUCT('Corner Bracket','Corner Bracket',
'LEGAL AND USAGE DISCLAIMER: this Data/Model is provided \X2\201C\X0\A
S IS\X2\201D\X0\ for informational and representational only. It is a 
geometric approximation and is NOT engineered, certified, or guarantee
d for dimensional accuracy, exact tolerances, or production-level prec
ision. Vendor disclaims all implied warranties including fitness for a
 particular purpose. DO NOT USE FOR DIRECT PHYSICAL MANUFACTURING, AUT
OMATED PRODUCTION, OR SAFETY-CRITICAL SYSTEMS without independent engi
neering verification and resolution of any design discrepancies.',(#7861));
#7873=PRESENTATION_STYLE_ASSIGNMENT((#7880));
#7880=SURFACE_STYLE_USAGE(.BOTH.,#7887);
#7887=SURFACE_SIDE_STYLE('',(#7894));
#7894=SURFACE_STYLE_FILL_AREA(#7901);
#7901=FILL_AREA_STYLE('Opaque(246,246,243)',(#7908));
#7908=FILL_AREA_STYLE_COLOUR('Opaque(246,246,243)',#7915);
#7915=COLOUR_RGB('Opaque(246,246,243)',0.964705882352941,0.964705882352941,
0.952941176470588);
ENDSEC;
END-ISO-10303-21;
